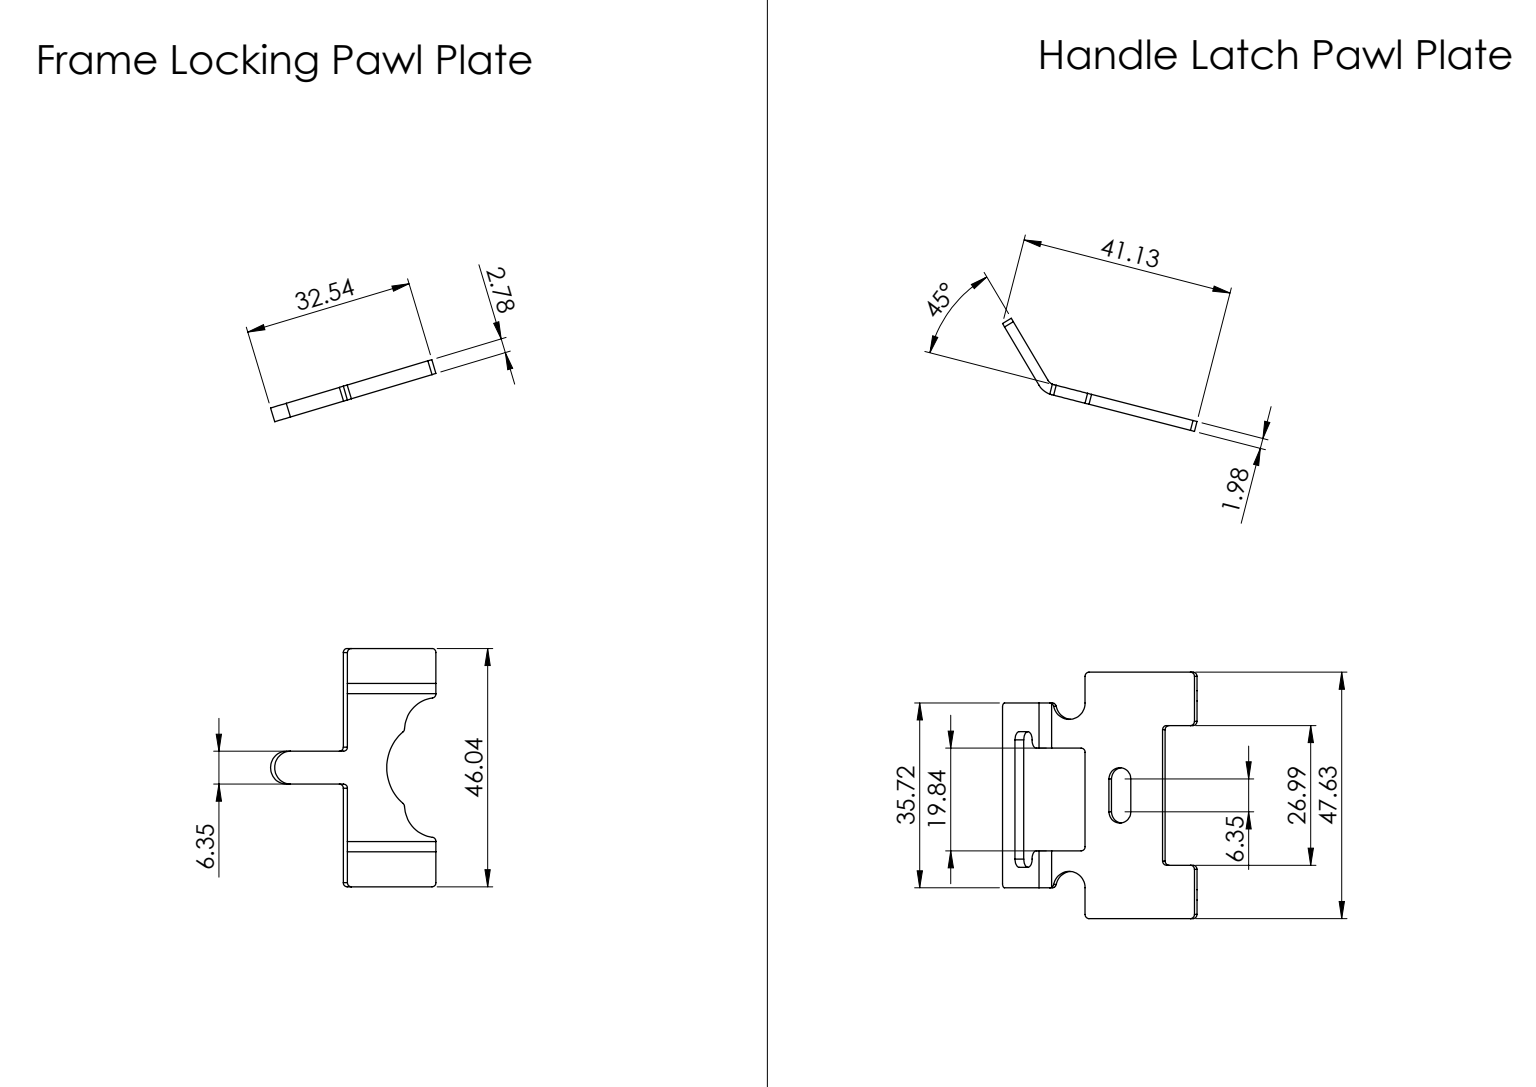
ISO-10303-21;
HEADER;
FILE_DESCRIPTION (('STEP AP214'),
    '1' );
FILE_NAME ('Frame Locking Pawl Plate.step',
    '2026-10-09T14:10:49',
    ( '' ),
    ( '' ),
    'SwSTEP 2.0',
    'SolidWorks 2026',
    '' );
FILE_SCHEMA (( 'AUTOMOTIVE_DESIGN' ));
ENDSEC;

DATA;
#12=VECTOR ( 'NONE', #9469, 1000.000000000000227 ) ;
#61=CARTESIAN_POINT ( 'NONE',  ( 14.43917063414567536, -6.754812500000002551, 2.343183994106907697 ) ) ;
#87=ORIENTED_EDGE ( 'NONE', *, *, #3995, .F. ) ;
#93=VERTEX_POINT ( 'NONE', #19156 ) ;
#123=DIRECTION ( 'NONE',  ( 0.2868778675745011220, 0.000000000000000000, 0.9579671649362034858 ) ) ;
#130=CARTESIAN_POINT ( 'NONE',  ( 13.67756757867809725, 20.23395749999999893, 2.571257636385987144 ) ) ;
#285=ORIENTED_EDGE ( 'NONE', *, *, #4081, .F. ) ;
#292=CARTESIAN_POINT ( 'NONE',  ( 29.98909767165928386, 30.50833916023545811, -5.214162619065493054 ) ) ;
#304=VERTEX_POINT ( 'NONE', #16295 ) ;
#353=DIRECTION ( 'NONE',  ( 0.000000000000000000, -1.000000000000000000, 0.000000000000000000 ) ) ;
#357=VECTOR ( 'NONE', #20266, 1000.000000000000000 ) ;
#367=VERTEX_POINT ( 'NONE', #5509 ) ;
#389=EDGE_CURVE ( 'NONE', #18438, #18286, #10607, .T. ) ;
#413=LINE ( 'NONE', #20514, #19877 ) ;
#419=EDGE_CURVE ( 'NONE', #13188, #14728, #15986, .T. ) ;
#453=ADVANCED_FACE ( 'NONE', ( #15932 ), #20761, .T. ) ;
#500=CARTESIAN_POINT ( 'NONE',  ( 13.67756757867809725, 38.48766750000000059, 2.571257636385987144 ) ) ;
#503=VECTOR ( 'NONE', #5511, 1000.000000000000227 ) ;
#522=CARTESIAN_POINT ( 'NONE',  ( 14.43917063414567536, 39.28268749999999443, 2.343183994106907697 ) ) ;
#539=VERTEX_POINT ( 'NONE', #21310 ) ;
#544=EDGE_CURVE ( 'NONE', #7495, #1968, #3265, .T. ) ;
#640=ORIENTED_EDGE ( 'NONE', *, *, #20179, .T. ) ;
#679=DIRECTION ( 'NONE',  ( 0.2868778675745011220, 0.000000000000000000, 0.9579671649362033747 ) ) ;
#697=LINE ( 'NONE', #19041, #16642 ) ;
#699=VERTEX_POINT ( 'NONE', #3620 ) ;
#749=ORIENTED_EDGE ( 'NONE', *, *, #21150, .T. ) ;
#760=DIRECTION ( 'NONE',  ( 0.000000000000000000, -1.000000000000000000, 0.000000000000000000 ) ) ;
#775=LINE ( 'NONE', #19445, #8515 ) ;
#847=CARTESIAN_POINT ( 'NONE',  ( 13.67756757867809725, -5.959792500000001603, 2.571257636385987144 ) ) ;
#868=ADVANCED_FACE ( 'NONE', ( #18966 ), #7371, .T. ) ;
#886=CARTESIAN_POINT ( 'NONE',  ( 29.98909767165928386, 39.28268749999999443, -5.214162619065493054 ) ) ;
#891=ORIENTED_EDGE ( 'NONE', *, *, #18599, .F. ) ;
#912=DIRECTION ( 'NONE',  ( 0.000000000000000000, 1.000000000000000000, 0.000000000000000000 ) ) ;
#944=DIRECTION ( 'NONE',  ( -0.2868778675745011220, 0.000000000000000000, -0.9579671649362034858 ) ) ;
#961=ORIENTED_EDGE ( 'NONE', *, *, #2073, .T. ) ;
#980=ORIENTED_EDGE ( 'NONE', *, *, #6673, .F. ) ;
#983=APPLICATION_CONTEXT ( 'automotive_design' ) ;
#996=CARTESIAN_POINT ( 'NONE',  ( 24.43309469626978725, 23.18727947754285879, -0.6496488801123181389 ) ) ;
#1024=LINE ( 'NONE', #4465, #19918 ) ;
#1049=FACE_OUTER_BOUND ( 'NONE', #12036, .T. ) ;
#1092=DIRECTION ( 'NONE',  ( 0.9579671649362032637, 0.000000000000000000, -0.2868778675745011775 ) ) ;
#1103=ORIENTED_EDGE ( 'NONE', *, *, #19401, .T. ) ;
#1104=DIRECTION ( 'NONE',  ( 0.9579671649362032637, 0.000000000000000000, -0.2868778675745010664 ) ) ;
#1115=EDGE_CURVE ( 'NONE', #20009, #20529, #13174, .T. ) ;
#1149=CARTESIAN_POINT ( 'NONE',  ( 29.22749461619170219, -6.754812500000002551, -4.986088976786413163 ) ) ;
#1157=ORIENTED_EDGE ( 'NONE', *, *, #8283, .T. ) ;
#1165=CARTESIAN_POINT ( 'NONE',  ( 30.78626241496060700, 30.50833916023545811, -2.552201779827368622 ) ) ;
#1191=ORIENTED_EDGE ( 'NONE', *, *, #8598, .F. ) ;
#1305=CARTESIAN_POINT ( 'NONE',  ( 13.67756757867809725, 0.001587500000000546807, 2.571257636385987144 ) ) ;
#1317=ORIENTED_EDGE ( 'NONE', *, *, #20399, .T. ) ;
#1328=CARTESIAN_POINT ( 'NONE',  ( 30.02465935949302533, 30.50833916023545811, -2.324128137548288731 ) ) ;
#1348=DIRECTION ( 'NONE',  ( 0.2868778675745011220, 0.000000000000000000, 0.9579671649362034858 ) ) ;
#1401=DIRECTION ( 'NONE',  ( 0.000000000000000000, -1.000000000000000000, 0.000000000000000000 ) ) ;
#1450=MECHANICAL_DESIGN_GEOMETRIC_PRESENTATION_REPRESENTATION('',(#2514),#7809);
#1483=AXIS2_PLACEMENT_3D ( 'NONE', #17356, #2200, #12384 ) ;
#1499=VERTEX_POINT ( 'NONE', #1305 ) ;
#1504=ORIENTED_EDGE ( 'NONE', *, *, #10980, .T. ) ;
#1583=DIRECTION ( 'NONE',  ( 0.2868778675745011220, 0.000000000000000000, 0.9579671649362034858 ) ) ;
#1586=ORIENTED_EDGE ( 'NONE', *, *, #5324, .F. ) ;
#1594=EDGE_LOOP ( 'NONE', ( #10062, #8009, #14700, #9478, #16584, #21246 ) ) ;
#1614=DIRECTION ( 'NONE',  ( 0.000000000000000000, 1.000000000000000000, 0.000000000000000000 ) ) ;
#1616=PLANE ( 'NONE',  #9906 ) ;
#1628=DIRECTION ( 'NONE',  ( 0.9579671649362032637, 0.000000000000000000, -0.2868778675745012885 ) ) ;
#1666=DIRECTION ( 'NONE',  ( -0.2868778675745011220, 0.000000000000000000, -0.9579671649362034858 ) ) ;
#1678=LINE ( 'NONE', #15312, #7096 ) ;
#1696=AXIS2_PLACEMENT_3D ( 'NONE', #16112, #944, #14450 ) ;
#1743=EDGE_LOOP ( 'NONE', ( #7465, #6376, #15613, #2042 ) ) ;
#1791=ORIENTED_EDGE ( 'NONE', *, *, #11880, .T. ) ;
#1847=DIRECTION ( 'NONE',  ( 0.000000000000000000, 1.000000000000000000, 0.000000000000000000 ) ) ;
#1883=EDGE_CURVE ( 'NONE', #20529, #15912, #413, .T. ) ;
#1968=VERTEX_POINT ( 'NONE', #9028 ) ;
#1980=CYLINDRICAL_SURFACE ( 'NONE', #5566, 8.929687500000001776 ) ;
#1986=ORIENTED_EDGE ( 'NONE', *, *, #8283, .F. ) ;
#1991=ORIENTED_EDGE ( 'NONE', *, *, #5836, .T. ) ;
#2037=DIRECTION ( 'NONE',  ( -0.9579671649362032637, 0.000000000000000000, 0.2868778675745010664 ) ) ;
#2041=VECTOR ( 'NONE', #20727, 1000.000000000000227 ) ;
#2042=ORIENTED_EDGE ( 'NONE', *, *, #14952, .T. ) ;
#2056=AXIS2_PLACEMENT_3D ( 'NONE', #11844, #18251, #3220 ) ;
#2073=EDGE_CURVE ( 'NONE', #18658, #16568, #9570, .T. ) ;
#2075=CARTESIAN_POINT ( 'NONE',  ( 12.91596452321051558, 20.23395749999999893, 2.799331278665067479 ) ) ;
#2131=FILL_AREA_STYLE ('',( #8988 ) ) ;
#2168=CARTESIAN_POINT ( 'NONE',  ( 2.651964239740473683, 19.43893749999999798, 5.873042593501262232 ) ) ;
#2182=EDGE_LOOP ( 'NONE', ( #7820, #21657, #6898, #18046 ) ) ;
#2200=DIRECTION ( 'NONE',  ( -0.2868778675745011220, 0.000000000000000000, -0.9579671649362034858 ) ) ;
#2230=CARTESIAN_POINT ( 'NONE',  ( 17.85969298310271114, 32.52628750000000224, 1.318856445756055873 ) ) ;
#2234=AXIS2_PLACEMENT_3D ( 'NONE', #14022, #2275, #17644 ) ;
#2244=VECTOR ( 'NONE', #14358, 1000.000000000000227 ) ;
#2254=ORIENTED_EDGE ( 'NONE', *, *, #6519, .T. ) ;
#2275=DIRECTION ( 'NONE',  ( 0.000000000000000000, 0.000000000000000000, 1.000000000000000000 ) ) ;
#2309=CARTESIAN_POINT ( 'NONE',  ( 14.43917063414567536, 39.28268749999999443, 2.343183994106907697 ) ) ;
#2314=EDGE_LOOP ( 'NONE', ( #18332, #4923, #10343, #5168 ) ) ;
#2324=CARTESIAN_POINT ( 'NONE',  ( 1.854799496439154316, 16.26393749999999727, 3.211081754263136911 ) ) ;
#2329=DIRECTION ( 'NONE',  ( -0.9579671649362030417, 0.000000000000000000, 0.2868778675745017326 ) ) ;
#2377=ORIENTED_EDGE ( 'NONE', *, *, #3048, .F. ) ;
#2406=CARTESIAN_POINT ( 'NONE',  ( 13.67756757867809725, 38.48766750000000059, 2.571257636385987144 ) ) ;
#2408=ORIENTED_EDGE ( 'NONE', *, *, #389, .F. ) ;
#2416=ORIENTED_EDGE ( 'NONE', *, *, #15750, .T. ) ;
#2471=SURFACE_STYLE_USAGE ( .BOTH. , #15984 ) ;
#2514=STYLED_ITEM ( 'NONE', ( #13999 ), #6428 ) ;
#2517=ORIENTED_EDGE ( 'NONE', *, *, #9221, .T. ) ;
#2553=AXIS2_PLACEMENT_3D ( 'NONE', #9600, #19557, #18127 ) ;
#2573=CARTESIAN_POINT ( 'NONE',  ( 30.78626241496060700, -5.959792500000001603, -2.552201779827368622 ) ) ;
#2602=EDGE_LOOP ( 'NONE', ( #11906, #1791, #11117, #1103 ) ) ;
#2617=ORIENTED_EDGE ( 'NONE', *, *, #8323, .F. ) ;
#2623=CARTESIAN_POINT ( 'NONE',  ( 29.03861462519914838, 16.26393749999999727, -4.929525984831418128 ) ) ;
#2642=ORIENTED_EDGE ( 'NONE', *, *, #15646, .F. ) ;
#2646=PLANE ( 'NONE',  #13935 ) ;
#2695=DIRECTION ( 'NONE',  ( 0.6050250551579484659, -0.7753173868113210077, -0.1811839737371541414 ) ) ;
#2707=CARTESIAN_POINT ( 'NONE',  ( 30.78626241496060700, 30.54508749999999750, -2.552201779827368622 ) ) ;
#2733=CARTESIAN_POINT ( 'NONE',  ( 1.854799496439154316, 19.43893749999999798, 3.211081754263136911 ) ) ;
#2741=EDGE_LOOP ( 'NONE', ( #14917, #640, #16235, #11591 ) ) ;
#2751=AXIS2_PLACEMENT_3D ( 'NONE', #1328, #21561, #13077 ) ;
#2752=EDGE_LOOP ( 'NONE', ( #2617, #17130, #21168, #2517, #13607, #11181 ) ) ;
#2754=CARTESIAN_POINT ( 'NONE',  ( 30.78626241496060700, 30.50833916023545811, -2.552201779827368622 ) ) ;
#2793=CYLINDRICAL_SURFACE ( 'NONE', #8442, 6.350000000000001421 ) ;
#2804=FACE_OUTER_BOUND ( 'NONE', #2847, .T. ) ;
#2834=VECTOR ( 'NONE', #18906, 1000.000000000000000 ) ;
#2843=LINE ( 'NONE', #2733, #12 ) ;
#2847=EDGE_LOOP ( 'NONE', ( #13729, #21082, #4101, #13970 ) ) ;
#2857=CARTESIAN_POINT ( 'NONE',  ( 12.91596452321051558, 12.29391749999999739, 2.799331278665067479 ) ) ;
#2875=CARTESIAN_POINT ( 'NONE',  ( 30.10940225190841701, 2.809619014187358932, -2.349505688218141319 ) ) ;
#2888=CARTESIAN_POINT ( 'NONE',  ( 29.98909767165928386, 38.48766750000000059, -5.214162619065493054 ) ) ;
#2895=CARTESIAN_POINT ( 'NONE',  ( 1.854799496439154316, 13.08893749999999834, 3.211081754263136911 ) ) ;
#2941=EDGE_LOOP ( 'NONE', ( #9817, #8604, #12640, #18611 ) ) ;
#2999=ADVANCED_FACE ( 'NONE', ( #11044 ), #2646, .T. ) ;
#3048=EDGE_CURVE ( 'NONE', #12509, #19832, #7231, .T. ) ;
#3169=VERTEX_POINT ( 'NONE', #8888 ) ;
#3182=ADVANCED_FACE ( 'NONE', ( #11587 ), #7010, .T. ) ;
#3220=DIRECTION ( 'NONE',  ( 0.9579671649362032637, 0.000000000000000000, -0.2868778675745011775 ) ) ;
#3233=FACE_OUTER_BOUND ( 'NONE', #1743, .T. ) ;
#3237=VECTOR ( 'NONE', #912, 1000.000000000000000 ) ;
#3265=CIRCLE ( 'NONE', #20890, 0.7950200000000005041 ) ;
#3291=FACE_OUTER_BOUND ( 'NONE', #2741, .T. ) ;
#3351=PLANE ( 'NONE',  #18829 ) ;
#3353=LINE ( 'NONE', #15082, #4579 ) ;
#3449=FACE_OUTER_BOUND ( 'NONE', #8597, .T. ) ;
#3511=ORIENTED_EDGE ( 'NONE', *, *, #20455, .T. ) ;
#3516=CARTESIAN_POINT ( 'NONE',  ( 12.11879977990919421, 19.43893749999999798, 0.1373704394269426865 ) ) ;
#3519=VERTEX_POINT ( 'NONE', #1149 ) ;
#3545=LINE ( 'NONE', #10282, #13496 ) ;
#3585=ADVANCED_FACE ( 'NONE', ( #18487 ), #20127, .F. ) ;
#3599=EDGE_LOOP ( 'NONE', ( #7691, #17588, #10865, #20840 ) ) ;
#3614=VECTOR ( 'NONE', #20424, 1000.000000000000000 ) ;
#3618=ORIENTED_EDGE ( 'NONE', *, *, #20772, .T. ) ;
#3620=CARTESIAN_POINT ( 'NONE',  ( 12.88040283537677588, 12.29391749999999739, -0.09070320285213756550 ) ) ;
#3624=LINE ( 'NONE', #13805, #21432 ) ;
#3636=ORIENTED_EDGE ( 'NONE', *, *, #13339, .F. ) ;
#3644=ORIENTED_EDGE ( 'NONE', *, *, #13978, .F. ) ;
#3653=CARTESIAN_POINT ( 'NONE',  ( 22.04181838752732148, 16.26393749999999727, 0.06645525512612464325 ) ) ;
#3656=ORIENTED_EDGE ( 'NONE', *, *, #15060, .T. ) ;
#3734=DIRECTION ( 'NONE',  ( 0.9579671649362032637, 0.000000000000000000, -0.2868778675745013440 ) ) ;
#3818=ORIENTED_EDGE ( 'NONE', *, *, #1115, .F. ) ;
#3826=CARTESIAN_POINT ( 'NONE',  ( 29.83577936850046441, 16.26393749999999727, -2.267565145593293696 ) ) ;
#3842=DIRECTION ( 'NONE',  ( 0.2868778675745011220, 0.000000000000000000, 0.9579671649362034858 ) ) ;
#3900=CIRCLE ( 'NONE', #18402, 0.7950200000000005041 ) ;
#3920=ORIENTED_EDGE ( 'NONE', *, *, #389, .T. ) ;
#3950=CARTESIAN_POINT ( 'NONE',  ( 12.91596452321051558, 19.43893749999999798, 2.799331278665067479 ) ) ;
#3951=DIRECTION ( 'NONE',  ( 0.9579671649362032637, 0.000000000000000000, -0.2868778675745010664 ) ) ;
#3960=ORIENTED_EDGE ( 'NONE', *, *, #4201, .F. ) ;
#3971=AXIS2_PLACEMENT_3D ( 'NONE', #19107, #7394, #14165 ) ;
#3995=EDGE_CURVE ( 'NONE', #4404, #11521, #17573, .T. ) ;
#4046=CARTESIAN_POINT ( 'NONE',  ( 12.88040283537677588, 20.23395749999999893, -0.09070320285213756550 ) ) ;
#4067=DIRECTION ( 'NONE',  ( -0.2868778675745010664, 0.000000000000000000, -0.9579671649362032637 ) ) ;
#4081=EDGE_CURVE ( 'NONE', #15859, #10888, #8991, .T. ) ;
#4101=ORIENTED_EDGE ( 'NONE', *, *, #6921, .T. ) ;
#4128=( NAMED_UNIT ( * ) SI_UNIT ( $, .STERADIAN. ) SOLID_ANGLE_UNIT ( ) );
#4131=CIRCLE ( 'NONE', #12241, 3.175000000000000711 ) ;
#4136=ADVANCED_FACE ( 'NONE', ( #14606 ), #21647, .T. ) ;
#4144=UNCERTAINTY_MEASURE_WITH_UNIT (LENGTH_MEASURE( 1.000000000000000082E-05 ), #9340, 'distance_accuracy_value', 'NONE');
#4146=CIRCLE ( 'NONE', #16510, 8.929687500000000000 ) ;
#4186=CIRCLE ( 'NONE', #2056, 0.7950200000000011702 ) ;
#4201=EDGE_CURVE ( 'NONE', #17126, #19423, #15035, .T. ) ;
#4238=ORIENTED_EDGE ( 'NONE', *, *, #18010, .F. ) ;
#4285=LINE ( 'NONE', #2406, #14814 ) ;
#4305=DIRECTION ( 'NONE',  ( -0.1065921516619563053, -0.9937903127262235348, 0.03192064434796804129 ) ) ;
#4329=VECTOR ( 'NONE', #20195, 1000.000000000000227 ) ;
#4353=ORIENTED_EDGE ( 'NONE', *, *, #10760, .T. ) ;
#4404=VERTEX_POINT ( 'NONE', #18434 ) ;
#4415=AXIS2_PLACEMENT_3D ( 'NONE', #13870, #18919, #353 ) ;
#4432=DIRECTION ( 'NONE',  ( 0.000000000000000000, 1.000000000000000000, 0.000000000000000000 ) ) ;
#4438=DIRECTION ( 'NONE',  ( -0.9579671649362033747, 0.000000000000000000, 0.2868778675745011220 ) ) ;
#4465=CARTESIAN_POINT ( 'NONE',  ( 12.11879977990919421, 19.43893749999999798, 0.1373704394269426865 ) ) ;
#4470=DIRECTION ( 'NONE',  ( 0.000000000000000000, 1.000000000000000000, 0.000000000000000000 ) ) ;
#4487=PLANE ( 'NONE',  #4539 ) ;
#4498=ORIENTED_EDGE ( 'NONE', *, *, #21150, .F. ) ;
#4518=CARTESIAN_POINT ( 'NONE',  ( 29.98909767165928386, -6.754812500000002551, -5.214162619065493054 ) ) ;
#4535=EDGE_CURVE ( 'NONE', #699, #15950, #5127, .T. ) ;
#4539=AXIS2_PLACEMENT_3D ( 'NONE', #9015, #11336, #8338 ) ;
#4543=LINE ( 'NONE', #19781, #12358 ) ;
#4574=LINE ( 'NONE', #19602, #14602 ) ;
#4579=VECTOR ( 'NONE', #13637, 1000.000000000000227 ) ;
#4584=VERTEX_POINT ( 'NONE', #522 ) ;
#4597=VERTEX_POINT ( 'NONE', #19604 ) ;
#4627=CARTESIAN_POINT ( 'NONE',  ( 23.15492293361681320, 8.724202693596797786, -3.167564836549936480 ) ) ;
#4652=AXIS2_PLACEMENT_3D ( 'NONE', #14182, #10736, #7305 ) ;
#4673=ORIENTED_EDGE ( 'NONE', *, *, #6673, .T. ) ;
#4682=DIRECTION ( 'NONE',  ( 0.2868778675745010664, 0.000000000000000000, 0.9579671649362032637 ) ) ;
#4707=EDGE_LOOP ( 'NONE', ( #3960, #4238, #8843, #749 ) ) ;
#4738=CYLINDRICAL_SURFACE ( 'NONE', #10361, 0.7950200000000005041 ) ;
#4753=ORIENTED_EDGE ( 'NONE', *, *, #9918, .T. ) ;
#4759=VERTEX_POINT ( 'NONE', #9756 ) ;
#4772=ORIENTED_EDGE ( 'NONE', *, *, #16413, .T. ) ;
#4774=DIRECTION ( 'NONE',  ( 0.000000000000000000, -1.000000000000000000, 0.000000000000000000 ) ) ;
#4810=DIRECTION ( 'NONE',  ( -0.2868778675745010664, 0.000000000000000000, -0.9579671649362032637 ) ) ;
#4898=EDGE_CURVE ( 'NONE', #699, #19423, #17273, .T. ) ;
#4919=CARTESIAN_POINT ( 'NONE',  ( 24.99127163628573456, 23.80367230640320031, 2.964528152719008158 ) ) ;
#4923=ORIENTED_EDGE ( 'NONE', *, *, #20455, .F. ) ;
#4958=ORIENTED_EDGE ( 'NONE', *, *, #4081, .T. ) ;
#5019=ORIENTED_EDGE ( 'NONE', *, *, #5849, .F. ) ;
#5022=AXIS2_PLACEMENT_3D ( 'NONE', #4919, #11559, #11458 ) ;
#5039=CARTESIAN_POINT ( 'NONE',  ( 30.78626241496060700, 2.019535839764540430, -2.552201779827368622 ) ) ;
#5042=CIRCLE ( 'NONE', #14600, 0.7950199999999993938 ) ;
#5089=CARTESIAN_POINT ( 'NONE',  ( 29.03861462519914838, 16.26393749999999727, -4.929525984831418128 ) ) ;
#5095=DIRECTION ( 'NONE',  ( -0.2868778675745010664, 0.000000000000000000, -0.9579671649362032637 ) ) ;
#5099=ORIENTED_EDGE ( 'NONE', *, *, #8046, .F. ) ;
#5127=CIRCLE ( 'NONE', #15398, 0.7950199999999993938 ) ;
#5168=ORIENTED_EDGE ( 'NONE', *, *, #6705, .F. ) ;
#5182=CARTESIAN_POINT ( 'NONE',  ( 24.71252020198295085, 8.768263569673496960, -0.7333271064221494884 ) ) ;
#5299=DIRECTION ( 'NONE',  ( 0.9579671649362032637, 0.000000000000000000, -0.2868778675745010664 ) ) ;
#5324=EDGE_CURVE ( 'NONE', #9688, #15950, #18352, .T. ) ;
#5353=DIRECTION ( 'NONE',  ( -0.9579671649362033747, 0.000000000000000000, 0.2868778675745011220 ) ) ;
#5379=AXIS2_PLACEMENT_3D ( 'NONE', #3826, #8677, #15451 ) ;
#5391=CARTESIAN_POINT ( 'NONE',  ( 14.43917063414567536, 38.48766750000000059, 2.343183994106907697 ) ) ;
#5404=DIRECTION ( 'NONE',  ( 0.9579671649362033747, 0.000000000000000000, -0.2868778675745010664 ) ) ;
#5437=CARTESIAN_POINT ( 'NONE',  ( 14.43917063414567536, -6.754812500000002551, 2.343183994106907697 ) ) ;
#5485=LINE ( 'NONE', #7161, #7416 ) ;
#5488=ORIENTED_EDGE ( 'NONE', *, *, #6705, .T. ) ;
#5509=CARTESIAN_POINT ( 'NONE',  ( 13.67756757867809725, -5.959792500000001603, 2.571257636385987144 ) ) ;
#5511=DIRECTION ( 'NONE',  ( -0.2868778675745010664, 0.000000000000000000, -0.9579671649362032637 ) ) ;
#5515=ORIENTED_EDGE ( 'NONE', *, *, #16413, .F. ) ;
#5539=DIRECTION ( 'NONE',  ( 0.9579671649362032637, 0.000000000000000000, -0.2868778675745010664 ) ) ;
#5546=DIRECTION ( 'NONE',  ( 0.2868778675745010664, 0.000000000000000000, 0.9579671649362032637 ) ) ;
#5555=ORIENTED_EDGE ( 'NONE', *, *, #17087, .T. ) ;
#5566=AXIS2_PLACEMENT_3D ( 'NONE', #5089, #8720, #5404 ) ;
#5639=VERTEX_POINT ( 'NONE', #19117 ) ;
#5676=AXIS2_PLACEMENT_3D ( 'NONE', #21844, #13355, #1614 ) ;
#5742=EDGE_CURVE ( 'NONE', #18438, #4597, #6077, .T. ) ;
#5780=ORIENTED_EDGE ( 'NONE', *, *, #11880, .F. ) ;
#5836=EDGE_CURVE ( 'NONE', #12549, #304, #20532, .T. ) ;
#5849=EDGE_CURVE ( 'NONE', #6840, #93, #20183, .T. ) ;
#5885=DIRECTION ( 'NONE',  ( 0.9579671649362033747, 0.000000000000000000, -0.2868778675745010664 ) ) ;
#6022=CYLINDRICAL_SURFACE ( 'NONE', #9479, 0.7950200000000003930 ) ;
#6077=CIRCLE ( 'NONE', #7848, 0.7950200000000011702 ) ;
#6081=ADVANCED_FACE ( 'NONE', ( #10112 ), #19843, .T. ) ;
#6106=ORIENTED_EDGE ( 'NONE', *, *, #6925, .T. ) ;
#6117=DIRECTION ( 'NONE',  ( 0.9579671649362033747, 0.000000000000000000, -0.2868778675745010664 ) ) ;
#6230=ORIENTED_EDGE ( 'NONE', *, *, #11251, .T. ) ;
#6244=LINE ( 'NONE', #6352, #10771 ) ;
#6260=ORIENTED_EDGE ( 'NONE', *, *, #4201, .T. ) ;
#6306=DIRECTION ( 'NONE',  ( 0.2868778675745011220, 0.000000000000000000, 0.9579671649362034858 ) ) ;
#6352=CARTESIAN_POINT ( 'NONE',  ( 29.22749461619170219, 39.28268749999999443, -4.986088976786413163 ) ) ;
#6376=ORIENTED_EDGE ( 'NONE', *, *, #19723, .F. ) ;
#6379=VECTOR ( 'NONE', #10460, 1000.000000000000227 ) ;
#6396=DIRECTION ( 'NONE',  ( 0.000000000000000000, -1.000000000000000000, 0.000000000000000000 ) ) ;
#6428=MANIFOLD_SOLID_BREP ( 'Stock-MAS-676-1', #9231 ) ;
#6448=AXIS2_PLACEMENT_3D ( 'NONE', #16744, #1583, #8327 ) ;
#6509=PRODUCT ( 'Frame Locking Pawl Plate', 'Frame Locking Pawl Plate', '', ( #20468 ) ) ;
#6519=EDGE_CURVE ( 'NONE', #18557, #3519, #697, .T. ) ;
#6562=PLANE ( 'NONE',  #7154 ) ;
#6588=ORIENTED_EDGE ( 'NONE', *, *, #544, .F. ) ;
#6599=ORIENTED_EDGE ( 'NONE', *, *, #3048, .T. ) ;
#6610=LINE ( 'NONE', #13593, #8886 ) ;
#6632=LINE ( 'NONE', #13622, #18426 ) ;
#6673=EDGE_CURVE ( 'NONE', #12549, #17651, #8204, .T. ) ;
#6700=CARTESIAN_POINT ( 'NONE',  ( 12.88040283537677588, -6.754812500000002551, -0.09070320285213756550 ) ) ;
#6703=ADVANCED_FACE ( 'NONE', ( #16925 ), #13633, .T. ) ;
#6705=EDGE_CURVE ( 'NONE', #7786, #17651, #16266, .T. ) ;
#6706=ADVANCED_FACE ( 'NONE', ( #3233 ), #16615, .T. ) ;
#6726=PLANE ( 'NONE',  #12969 ) ;
#6822=CIRCLE ( 'NONE', #10718, 0.7950199999999993938 ) ;
#6840=VERTEX_POINT ( 'NONE', #13737 ) ;
#6852=ADVANCED_FACE ( 'NONE', ( #20668 ), #9063, .T. ) ;
#6885=DIRECTION ( 'NONE',  ( 0.000000000000000000, -1.000000000000000000, 0.000000000000000000 ) ) ;
#6897=DIRECTION ( 'NONE',  ( 0.000000000000000000, 1.000000000000000000, 0.000000000000000000 ) ) ;
#6898=ORIENTED_EDGE ( 'NONE', *, *, #15391, .F. ) ;
#6921=EDGE_CURVE ( 'NONE', #7865, #6840, #15407, .T. ) ;
#6925=EDGE_CURVE ( 'NONE', #10936, #5639, #14073, .T. ) ;
#6949=ADVANCED_FACE ( 'NONE', ( #10410 ), #17152, .T. ) ;
#6962=LINE ( 'NONE', #20004, #11377 ) ;
#7010=PLANE ( 'NONE',  #16065 ) ;
#7042=EDGE_CURVE ( 'NONE', #539, #7495, #17819, .T. ) ;
#7096=VECTOR ( 'NONE', #15195, 1000.000000000000227 ) ;
#7132=AXIS2_PLACEMENT_3D ( 'NONE', #3653, #13838, #17141 ) ;
#7137=DIRECTION ( 'NONE',  ( -0.2868778675745011220, 0.000000000000000000, -0.9579671649362034858 ) ) ;
#7148=LINE ( 'NONE', #15230, #16299 ) ;
#7154=AXIS2_PLACEMENT_3D ( 'NONE', #18068, #9542, #14665 ) ;
#7161=CARTESIAN_POINT ( 'NONE',  ( 12.11879977990919421, 13.08893749999999834, 0.1373704394269426865 ) ) ;
#7207=ORIENTED_EDGE ( 'NONE', *, *, #18883, .F. ) ;
#7231=CIRCLE ( 'NONE', #19574, 6.350000000000002309 ) ;
#7262=ORIENTED_EDGE ( 'NONE', *, *, #15391, .T. ) ;
#7305=DIRECTION ( 'NONE',  ( 0.9564948366894089338, 0.05542109139015086172, -0.2864369564417716951 ) ) ;
#7322=FACE_OUTER_BOUND ( 'NONE', #1594, .T. ) ;
#7350=ORIENTED_EDGE ( 'NONE', *, *, #19779, .F. ) ;
#7359=DIRECTION ( 'NONE',  ( 0.2868778675745011220, 0.000000000000000000, 0.9579671649362033747 ) ) ;
#7371=PLANE ( 'NONE',  #17029 ) ;
#7394=DIRECTION ( 'NONE',  ( -0.2868778675745011220, 0.000000000000000000, -0.9579671649362034858 ) ) ;
#7407=DIRECTION ( 'NONE',  ( 0.000000000000000000, 1.000000000000000000, 0.000000000000000000 ) ) ;
#7416=VECTOR ( 'NONE', #10244, 1000.000000000000227 ) ;
#7465=ORIENTED_EDGE ( 'NONE', *, *, #5742, .F. ) ;
#7495=VERTEX_POINT ( 'NONE', #19186 ) ;
#7501=ORIENTED_EDGE ( 'NONE', *, *, #13815, .F. ) ;
#7557=CARTESIAN_POINT ( 'NONE',  ( 29.98909767165928386, 2.019535839764540430, -5.214162619065493054 ) ) ;
#7564=EDGE_LOOP ( 'NONE', ( #14812, #18530, #3818, #4353 ) ) ;
#7577=ORIENTED_EDGE ( 'NONE', *, *, #15750, .F. ) ;
#7589=CARTESIAN_POINT ( 'NONE',  ( 12.11879977990919421, 13.08893749999999834, 0.1373704394269426865 ) ) ;
#7633=DIRECTION ( 'NONE',  ( 0.2868778675745010664, 0.000000000000000000, 0.9579671649362032637 ) ) ;
#7666=DIRECTION ( 'NONE',  ( 0.2868778675745011220, 0.000000000000000000, 0.9579671649362034858 ) ) ;
#7691=ORIENTED_EDGE ( 'NONE', *, *, #9143, .T. ) ;
#7704=ORIENTED_EDGE ( 'NONE', *, *, #4898, .T. ) ;
#7738=ORIENTED_EDGE ( 'NONE', *, *, #8968, .T. ) ;
#7741=VECTOR ( 'NONE', #8594, 1000.000000000000227 ) ;
#7786=VERTEX_POINT ( 'NONE', #16342 ) ;
#7802=VECTOR ( 'NONE', #9794, 1000.000000000000000 ) ;
#7809=( GEOMETRIC_REPRESENTATION_CONTEXT ( 3 ) GLOBAL_UNCERTAINTY_ASSIGNED_CONTEXT ( ( #12116 ) ) GLOBAL_UNIT_ASSIGNED_CONTEXT ( ( #10539, #17177, #4128 ) ) REPRESENTATION_CONTEXT ( 'NONE', 'WORKASPACE' ) );
#7820=ORIENTED_EDGE ( 'NONE', *, *, #12450, .T. ) ;
#7830=AXIS2_PLACEMENT_3D ( 'NONE', #8160, #14938, #1628 ) ;
#7832=ORIENTED_EDGE ( 'NONE', *, *, #6921, .F. ) ;
#7848=AXIS2_PLACEMENT_3D ( 'NONE', #16366, #21427, #1092 ) ;
#7865=VERTEX_POINT ( 'NONE', #21626 ) ;
#7960=EDGE_CURVE ( 'NONE', #5639, #14728, #19153, .T. ) ;
#8009=ORIENTED_EDGE ( 'NONE', *, *, #12944, .T. ) ;
#8017=ORIENTED_EDGE ( 'NONE', *, *, #5836, .F. ) ;
#8044=DIRECTION ( 'NONE',  ( -0.2868778675745011220, 0.000000000000000000, -0.9579671649362034858 ) ) ;
#8046=EDGE_CURVE ( 'NONE', #9688, #539, #10121, .T. ) ;
#8051=DIRECTION ( 'NONE',  ( 0.000000000000000000, 1.000000000000000000, 0.000000000000000000 ) ) ;
#8077=ORIENTED_EDGE ( 'NONE', *, *, #419, .F. ) ;
#8100=CARTESIAN_POINT ( 'NONE',  ( 30.78626241496060700, 38.48766750000000059, -2.552201779827368622 ) ) ;
#8116=AXIS2_PLACEMENT_3D ( 'NONE', #16863, #7137, #13906 ) ;
#8123=VECTOR ( 'NONE', #15838, 1000.000000000000227 ) ;
#8152=CARTESIAN_POINT ( 'NONE',  ( 12.88040283537677588, 39.28268749999999443, -0.09070320285213756550 ) ) ;
#8157=ORIENTED_EDGE ( 'NONE', *, *, #9944, .F. ) ;
#8160=CARTESIAN_POINT ( 'NONE',  ( 11.07961582054159244, 12.29391749999999739, -3.332761710603877159 ) ) ;
#8204=LINE ( 'NONE', #11853, #14509 ) ;
#8271=LINE ( 'NONE', #21757, #4329 ) ;
#8283=EDGE_CURVE ( 'NONE', #19832, #10623, #9941, .T. ) ;
#8292=LINE ( 'NONE', #15064, #14421 ) ;
#8323=EDGE_CURVE ( 'NONE', #1499, #3169, #3545, .T. ) ;
#8327=DIRECTION ( 'NONE',  ( 0.9579671649362033747, 0.000000000000000000, -0.2868778675745011775 ) ) ;
#8338=DIRECTION ( 'NONE',  ( -0.2868778675745010664, 0.000000000000000000, -0.9579671649362032637 ) ) ;
#8339=LINE ( 'NONE', #13440, #20986 ) ;
#8374=ORIENTED_EDGE ( 'NONE', *, *, #17598, .T. ) ;
#8390=EDGE_CURVE ( 'NONE', #16118, #12232, #775, .T. ) ;
#8405=CARTESIAN_POINT ( 'NONE',  ( 21.24465364422600189, 16.26393749999999727, -2.595505584112000275 ) ) ;
#8416=CARTESIAN_POINT ( 'NONE',  ( 12.88040283537677588, 12.29391749999999739, -0.09070320285213756550 ) ) ;
#8442=AXIS2_PLACEMENT_3D ( 'NONE', #9529, #9197, #5885 ) ;
#8486=DIRECTION ( 'NONE',  ( 0.000000000000000000, 1.000000000000000000, 0.000000000000000000 ) ) ;
#8515=VECTOR ( 'NONE', #11059, 1000.000000000000000 ) ;
#8519=CARTESIAN_POINT ( 'NONE',  ( 31.06384331886062711, 2.019535839764540430, 1.146004012482531476 ) ) ;
#8594=DIRECTION ( 'NONE',  ( -0.9579671649362032637, 0.000000000000000000, 0.2868778675745010664 ) ) ;
#8597=EDGE_LOOP ( 'NONE', ( #8374, #2408, #8599, #7350, #12565, #20201, #4958, #891, #21710, #17751, #6230, #18622, #6260, #13138, #11604, #1586, #15759, #10248, #5488, #980, #1991, #9121 ) ) ;
#8598=EDGE_CURVE ( 'NONE', #4584, #4404, #17016, .T. ) ;
#8599=ORIENTED_EDGE ( 'NONE', *, *, #5742, .T. ) ;
#8602=DIRECTION ( 'NONE',  ( 0.2868778675745011220, 0.000000000000000000, 0.9579671649362034858 ) ) ;
#8604=ORIENTED_EDGE ( 'NONE', *, *, #11830, .T. ) ;
#8676=CARTESIAN_POINT ( 'NONE',  ( 30.02465935949302533, 2.019535839764540430, -2.324128137548288731 ) ) ;
#8677=DIRECTION ( 'NONE',  ( -0.2868778675745011220, 0.000000000000000000, -0.9579671649362034858 ) ) ;
#8720=DIRECTION ( 'NONE',  ( 0.2868778675745011220, 0.000000000000000000, 0.9579671649362034858 ) ) ;
#8733=CARTESIAN_POINT ( 'NONE',  ( 12.88040283537677588, 13.08893749999999834, -0.09070320285213756550 ) ) ;
#8756=ORIENTED_EDGE ( 'NONE', *, *, #6925, .F. ) ;
#8772=FACE_OUTER_BOUND ( 'NONE', #12318, .T. ) ;
#8843=ORIENTED_EDGE ( 'NONE', *, *, #17042, .F. ) ;
#8886=VECTOR ( 'NONE', #6396, 1000.000000000000000 ) ;
#8888=CARTESIAN_POINT ( 'NONE',  ( 30.78626241496060700, 0.001587500000000546807, -2.552201779827368622 ) ) ;
#8907=VECTOR ( 'NONE', #20620, 1000.000000000000227 ) ;
#8913=DIRECTION ( 'NONE',  ( 0.2868778675745011220, 0.000000000000000000, 0.9579671649362033747 ) ) ;
#8960=CARTESIAN_POINT ( 'NONE',  ( 24.71252020198295085, 23.75961143032650114, -0.7333271064221494884 ) ) ;
#8968=EDGE_CURVE ( 'NONE', #1968, #20661, #9578, .T. ) ;
#8988=FILL_AREA_STYLE_COLOUR ( '', #19454 ) ;
#8991=CIRCLE ( 'NONE', #16437, 0.7950200000000003930 ) ;
#9013=ORIENTED_EDGE ( 'NONE', *, *, #544, .T. ) ;
#9015=CARTESIAN_POINT ( 'NONE',  ( 1.854799496439154316, 13.08893749999999834, 3.211081754263136911 ) ) ;
#9028=CARTESIAN_POINT ( 'NONE',  ( 13.67756757867809725, 12.29391749999999739, 2.571257636385987144 ) ) ;
#9029=DIRECTION ( 'NONE',  ( -0.9564948366894091558, 0.05542109139015080621, 0.2864369564417710845 ) ) ;
#9058=DIRECTION ( 'NONE',  ( 0.2868778675745011220, 0.000000000000000000, 0.9579671649362034858 ) ) ;
#9063=CYLINDRICAL_SURFACE ( 'NONE', #12374, 0.7950199999999996159 ) ;
#9096=ADVANCED_FACE ( 'NONE', ( #3291 ), #1616, .T. ) ;
#9113=DIRECTION ( 'NONE',  ( 0.9579671649362032637, 0.000000000000000000, -0.2868778675745010664 ) ) ;
#9121=ORIENTED_EDGE ( 'NONE', *, *, #16069, .F. ) ;
#9143=EDGE_CURVE ( 'NONE', #10936, #20661, #7148, .T. ) ;
#9197=DIRECTION ( 'NONE',  ( 0.2868778675745011220, 0.000000000000000000, 0.9579671649362034858 ) ) ;
#9221=EDGE_CURVE ( 'NONE', #13909, #18557, #11796, .T. ) ;
#9231=CLOSED_SHELL ( 'NONE', ( #21826, #12597, #6852, #3182, #3585, #12612, #20119, #10996, #19671, #6949, #17071, #9096, #13483, #4136, #6703, #14723, #10981, #10004, #6081, #21521, #6706, #2999, #453, #16679, #868, #19211, #9352, #20616 ) ) ;
#9264=DIRECTION ( 'NONE',  ( -0.2868778675745011220, 0.000000000000000000, -0.9579671649362034858 ) ) ;
#9268=EDGE_CURVE ( 'NONE', #17651, #21745, #12007, .T. ) ;
#9291=DIRECTION ( 'NONE',  ( 0.2868778675745011220, 0.000000000000000000, 0.9579671649362034858 ) ) ;
#9329=CARTESIAN_POINT ( 'NONE',  ( 12.11879977990919421, 12.29391749999999739, 0.1373704394269426865 ) ) ;
#9340=( LENGTH_UNIT ( ) NAMED_UNIT ( * ) SI_UNIT ( .MILLI., .METRE. ) );
#9352=ADVANCED_FACE ( 'NONE', ( #12570 ), #15896, .T. ) ;
#9354=AXIS2_PLACEMENT_3D ( 'NONE', #19870, #8044, #16145 ) ;
#9469=DIRECTION ( 'NONE',  ( 0.2868778675745010664, 0.000000000000000000, 0.9579671649362032637 ) ) ;
#9478=ORIENTED_EDGE ( 'NONE', *, *, #13978, .T. ) ;
#9479=AXIS2_PLACEMENT_3D ( 'NONE', #12796, #19619, #12909 ) ;
#9495=CARTESIAN_POINT ( 'NONE',  ( 12.88040283537677588, 38.48766750000000059, -0.09070320285213756550 ) ) ;
#9525=CIRCLE ( 'NONE', #17292, 3.175000000000000711 ) ;
#9529=CARTESIAN_POINT ( 'NONE',  ( 29.98909767165928386, 9.120187499999998337, -5.214162619065493054 ) ) ;
#9542=DIRECTION ( 'NONE',  ( 0.2868778675745011220, 0.000000000000000000, 0.9579671649362033747 ) ) ;
#9570=LINE ( 'NONE', #16341, #2244 ) ;
#9578=LINE ( 'NONE', #13257, #7802 ) ;
#9600=CARTESIAN_POINT ( 'NONE',  ( 13.64200589084435578, 38.48766750000000059, -0.3187768451312169571 ) ) ;
#9688=VERTEX_POINT ( 'NONE', #11773 ) ;
#9702=DIRECTION ( 'NONE',  ( 0.000000000000000000, 1.000000000000000000, 0.000000000000000000 ) ) ;
#9756=CARTESIAN_POINT ( 'NONE',  ( 24.43309469626978725, 23.18727947754285879, -0.6496488801123181389 ) ) ;
#9794=DIRECTION ( 'NONE',  ( 0.000000000000000000, -1.000000000000000000, 0.000000000000000000 ) ) ;
#9817=ORIENTED_EDGE ( 'NONE', *, *, #16520, .F. ) ;
#9821=ORIENTED_EDGE ( 'NONE', *, *, #9268, .T. ) ;
#9841=ORIENTED_EDGE ( 'NONE', *, *, #8390, .F. ) ;
#9845=DIRECTION ( 'NONE',  ( -0.2868778675745011220, 0.000000000000000000, -0.9579671649362034858 ) ) ;
#9853=DIRECTION ( 'NONE',  ( 0.9579671649362033747, 0.000000000000000000, -0.2868778675745006779 ) ) ;
#9906=AXIS2_PLACEMENT_3D ( 'NONE', #6700, #13915, #20494 ) ;
#9918=EDGE_CURVE ( 'NONE', #17422, #16118, #16860, .T. ) ;
#9941=CIRCLE ( 'NONE', #4652, 0.7950199999999990608 ) ;
#9944=EDGE_CURVE ( 'NONE', #10623, #15859, #8292, .T. ) ;
#9955=LINE ( 'NONE', #11733, #3614 ) ;
#9985=LINE ( 'NONE', #14770, #12401 ) ;
#10004=ADVANCED_FACE ( 'NONE', ( #15605 ), #1980, .F. ) ;
#10062=ORIENTED_EDGE ( 'NONE', *, *, #15494, .T. ) ;
#10079=CARTESIAN_POINT ( 'NONE',  ( 12.11879977990919421, 20.23395749999999893, 0.1373704394269426865 ) ) ;
#10112=FACE_OUTER_BOUND ( 'NONE', #13240, .T. ) ;
#10121=LINE ( 'NONE', #16867, #19129 ) ;
#10183=DIRECTION ( 'NONE',  ( 0.9579671649362032637, 0.000000000000000000, -0.2868778675745010664 ) ) ;
#10201=ORIENTED_EDGE ( 'NONE', *, *, #9143, .F. ) ;
#10207=( NAMED_UNIT ( * ) SI_UNIT ( $, .STERADIAN. ) SOLID_ANGLE_UNIT ( ) );
#10235=ORIENTED_EDGE ( 'NONE', *, *, #14170, .F. ) ;
#10244=DIRECTION ( 'NONE',  ( 0.2868778675745010664, 0.000000000000000000, 0.9579671649362032637 ) ) ;
#10248=ORIENTED_EDGE ( 'NONE', *, *, #11830, .F. ) ;
#10260=ORIENTED_EDGE ( 'NONE', *, *, #16069, .T. ) ;
#10282=CARTESIAN_POINT ( 'NONE',  ( 26.41404040124396602, 0.001587500000000546807, -1.242873262350622010 ) ) ;
#10312=CIRCLE ( 'NONE', #19479, 6.350000000000005862 ) ;
#10343=ORIENTED_EDGE ( 'NONE', *, *, #9268, .F. ) ;
#10361=AXIS2_PLACEMENT_3D ( 'NONE', #11070, #17826, #1401 ) ;
#10391=DIRECTION ( 'NONE',  ( -0.2868778675745010664, 0.000000000000000000, -0.9579671649362032637 ) ) ;
#10410=FACE_OUTER_BOUND ( 'NONE', #13168, .T. ) ;
#10456=DIRECTION ( 'NONE',  ( 0.2868778675745011220, 0.000000000000000000, 0.9579671649362034858 ) ) ;
#10460=DIRECTION ( 'NONE',  ( 0.9579671649362032637, 0.000000000000000000, -0.2868778675745010664 ) ) ;
#10474=CARTESIAN_POINT ( 'NONE',  ( 29.98909767165928386, 23.40768749999999798, -5.214162619065493054 ) ) ;
#10492=CARTESIAN_POINT ( 'NONE',  ( 29.98909767165928386, 30.50833916023545811, -5.214162619065493054 ) ) ;
#10539=( LENGTH_UNIT ( ) NAMED_UNIT ( * ) SI_UNIT ( .MILLI., .METRE. ) );
#10560=DIRECTION ( 'NONE',  ( 0.9579671649362033747, 0.000000000000000000, -0.2868778675745006779 ) ) ;
#10585=CARTESIAN_POINT ( 'NONE',  ( 24.71252020198295085, 8.768263569673496960, -0.7333271064221494884 ) ) ;
#10607=LINE ( 'NONE', #10492, #16676 ) ;
#10623=VERTEX_POINT ( 'NONE', #20671 ) ;
#10718=AXIS2_PLACEMENT_3D ( 'NONE', #12735, #9291, #19459 ) ;
#10736=DIRECTION ( 'NONE',  ( 0.2868778675745011220, 0.000000000000000000, 0.9579671649362034858 ) ) ;
#10760=EDGE_CURVE ( 'NONE', #20009, #18286, #19572, .T. ) ;
#10771=VECTOR ( 'NONE', #19621, 1000.000000000000227 ) ;
#10808=ORIENTED_EDGE ( 'NONE', *, *, #13339, .T. ) ;
#10810=DIRECTION ( 'NONE',  ( 0.000000000000000000, -1.000000000000000000, 0.000000000000000000 ) ) ;
#10829=PLANE ( 'NONE',  #7132 ) ;
#10837=PLANE ( 'NONE',  #20700 ) ;
#10865=ORIENTED_EDGE ( 'NONE', *, *, #8323, .T. ) ;
#10885=( GEOMETRIC_REPRESENTATION_CONTEXT ( 3 ) GLOBAL_UNCERTAINTY_ASSIGNED_CONTEXT ( ( #4144 ) ) GLOBAL_UNIT_ASSIGNED_CONTEXT ( ( #9340, #20254, #10207 ) ) REPRESENTATION_CONTEXT ( 'NONE', 'WORKASPACE' ) );
#10888=VERTEX_POINT ( 'NONE', #10896 ) ;
#10896=CARTESIAN_POINT ( 'NONE',  ( 23.91535545868163126, 8.768263569673496960, -3.395287945660274254 ) ) ;
#10936=VERTEX_POINT ( 'NONE', #12676 ) ;
#10980=EDGE_CURVE ( 'NONE', #7865, #17422, #16558, .T. ) ;
#10981=ADVANCED_FACE ( 'NONE', ( #21167 ), #6022, .T. ) ;
#10993=PRODUCT_DEFINITION_CONTEXT ( 'detailed design', #983, 'design' ) ;
#10996=ADVANCED_FACE ( 'NONE', ( #1049 ), #4487, .T. ) ;
#11010=ORIENTED_EDGE ( 'NONE', *, *, #8390, .T. ) ;
#11018=SHAPE_REPRESENTATION ( 'Frame Locking Pawl Plate', ( #2234 ), #10885 ) ;
#11044=FACE_OUTER_BOUND ( 'NONE', #11878, .T. ) ;
#11046=DIRECTION ( 'NONE',  ( -0.2868778675745011220, 0.000000000000000000, -0.9579671649362034858 ) ) ;
#11059=DIRECTION ( 'NONE',  ( 0.000000000000000000, 1.000000000000000000, 0.000000000000000000 ) ) ;
#11070=CARTESIAN_POINT ( 'NONE',  ( 15.47835459351327714, -5.959792500000001603, 5.813316144137728791 ) ) ;
#11117=ORIENTED_EDGE ( 'NONE', *, *, #15060, .F. ) ;
#11157=DIRECTION ( 'NONE',  ( 0.9564948366894089338, -0.05542109139015086172, -0.2864369564417716951 ) ) ;
#11181=ORIENTED_EDGE ( 'NONE', *, *, #14170, .T. ) ;
#11209=FACE_OUTER_BOUND ( 'NONE', #2752, .T. ) ;
#11248=PRODUCT_DEFINITION_FORMATION_WITH_SPECIFIED_SOURCE ( 'ANY', '', #6509, .NOT_KNOWN. ) ;
#11250=EDGE_LOOP ( 'NONE', ( #12932, #10260, #7577, #3644 ) ) ;
#11251=EDGE_CURVE ( 'NONE', #16568, #3519, #4186, .T. ) ;
#11277=CIRCLE ( 'NONE', #16921, 0.7950200000000010592 ) ;
#11324=ORIENTED_EDGE ( 'NONE', *, *, #15646, .T. ) ;
#11328=DIRECTION ( 'NONE',  ( 0.9579671649362032637, 0.000000000000000000, -0.2868778675745010664 ) ) ;
#11336=DIRECTION ( 'NONE',  ( 0.000000000000000000, -1.000000000000000000, -0.000000000000000000 ) ) ;
#11372=CARTESIAN_POINT ( 'NONE',  ( 30.78626241496060700, 9.120187499999998337, -2.552201779827368622 ) ) ;
#11377=VECTOR ( 'NONE', #5095, 1000.000000000000227 ) ;
#11424=CARTESIAN_POINT ( 'NONE',  ( 29.98909767165928386, -5.959792500000001603, -5.214162619065493054 ) ) ;
#11439=ORIENTED_EDGE ( 'NONE', *, *, #7960, .F. ) ;
#11458=DIRECTION ( 'NONE',  ( 0.9564948366894089338, -0.05542109139015086172, -0.2864369564417716951 ) ) ;
#11476=DIRECTION ( 'NONE',  ( -0.2868778675745010664, 0.000000000000000000, -0.9579671649362032637 ) ) ;
#11478=AXIS2_PLACEMENT_3D ( 'NONE', #4518, #12832, #16254 ) ;
#11521=VERTEX_POINT ( 'NONE', #15044 ) ;
#11559=DIRECTION ( 'NONE',  ( -0.2868778675745011220, 0.000000000000000000, -0.9579671649362034858 ) ) ;
#11587=FACE_OUTER_BOUND ( 'NONE', #20533, .T. ) ;
#11591=ORIENTED_EDGE ( 'NONE', *, *, #9221, .F. ) ;
#11604=ORIENTED_EDGE ( 'NONE', *, *, #4535, .T. ) ;
#11666=AXIS2_PLACEMENT_3D ( 'NONE', #18260, #1666, #18364 ) ;
#11689=ORIENTED_EDGE ( 'NONE', *, *, #11251, .F. ) ;
#11733=CARTESIAN_POINT ( 'NONE',  ( 13.67756757867809725, 12.29391749999999739, 2.571257636385987144 ) ) ;
#11747=DIRECTION ( 'NONE',  ( 0.000000000000000000, -1.000000000000000000, 0.000000000000000000 ) ) ;
#11773=CARTESIAN_POINT ( 'NONE',  ( 1.854799496439154316, 13.08893749999999834, 3.211081754263136911 ) ) ;
#11796=LINE ( 'NONE', #61, #6379 ) ;
#11830=EDGE_CURVE ( 'NONE', #7786, #13109, #20297, .T. ) ;
#11837=DIRECTION ( 'NONE',  ( -0.2868778675745010664, 0.000000000000000000, -0.9579671649362032637 ) ) ;
#11844=CARTESIAN_POINT ( 'NONE',  ( 29.22749461619170219, -5.959792500000001603, -4.986088976786413163 ) ) ;
#11853=CARTESIAN_POINT ( 'NONE',  ( 12.88040283537677588, 38.48766750000000059, -0.09070320285213756550 ) ) ;
#11878=EDGE_LOOP ( 'NONE', ( #20937, #21634, #21638, #9841, #13781, #3920 ) ) ;
#11880=EDGE_CURVE ( 'NONE', #11521, #21727, #4285, .T. ) ;
#11906=ORIENTED_EDGE ( 'NONE', *, *, #15494, .F. ) ;
#11998=CARTESIAN_POINT ( 'NONE',  ( 30.78626241496060700, 32.52628750000000224, -2.552201779827368622 ) ) ;
#12007=LINE ( 'NONE', #18738, #15553 ) ;
#12029=EDGE_LOOP ( 'NONE', ( #18222, #16718, #19009, #20087 ) ) ;
#12036=EDGE_LOOP ( 'NONE', ( #17607, #20144, #5099, #18158 ) ) ;
#12093=FACE_OUTER_BOUND ( 'NONE', #2182, .T. ) ;
#12116=UNCERTAINTY_MEASURE_WITH_UNIT (LENGTH_MEASURE( 1.000000000000000082E-05 ), #10539, 'distance_accuracy_value', 'NONE');
#12232=VERTEX_POINT ( 'NONE', #2707 ) ;
#12233=CARTESIAN_POINT ( 'NONE',  ( 30.78626241496060700, 38.48766750000000059, -2.552201779827368622 ) ) ;
#12241=AXIS2_PLACEMENT_3D ( 'NONE', #2324, #9058, #4432 ) ;
#12268=DIRECTION ( 'NONE',  ( 0.000000000000000000, 1.000000000000000000, 0.000000000000000000 ) ) ;
#12285=ORIENTED_EDGE ( 'NONE', *, *, #2073, .F. ) ;
#12300=CARTESIAN_POINT ( 'NONE',  ( 29.98909767165928386, 9.120187499999998337, -5.214162619065493054 ) ) ;
#12312=SHAPE_DEFINITION_REPRESENTATION ( #14096, #11018 ) ;
#12318=EDGE_LOOP ( 'NONE', ( #11689, #12285, #7207, #2254 ) ) ;
#12349=ORIENTED_EDGE ( 'NONE', *, *, #18262, .T. ) ;
#12358=VECTOR ( 'NONE', #21120, 1000.000000000000227 ) ;
#12374=AXIS2_PLACEMENT_3D ( 'NONE', #20555, #19011, #2329 ) ;
#12384=DIRECTION ( 'NONE',  ( 0.1065921516619544457, 0.9937903127262237568, -0.03192064434796771516 ) ) ;
#12401=VECTOR ( 'NONE', #16742, 1000.000000000000227 ) ;
#12419=DIRECTION ( 'NONE',  ( -0.2868778675745011220, 0.000000000000000000, -0.9579671649362034858 ) ) ;
#12431=FACE_OUTER_BOUND ( 'NONE', #20159, .T. ) ;
#12435=SURFACE_STYLE_FILL_AREA ( #2131 ) ;
#12450=EDGE_CURVE ( 'NONE', #13109, #9688, #4131, .T. ) ;
#12491=VECTOR ( 'NONE', #11476, 1000.000000000000227 ) ;
#12509=VERTEX_POINT ( 'NONE', #2875 ) ;
#12549=VERTEX_POINT ( 'NONE', #9495 ) ;
#12565=ORIENTED_EDGE ( 'NONE', *, *, #5849, .T. ) ;
#12570=FACE_OUTER_BOUND ( 'NONE', #3599, .T. ) ;
#12597=ADVANCED_FACE ( 'NONE', ( #16054 ), #10837, .T. ) ;
#12612=ADVANCED_FACE ( 'NONE', ( #15946 ), #6726, .T. ) ;
#12634=CARTESIAN_POINT ( 'NONE',  ( 22.04181838752732148, 16.26393749999999727, 0.06645525512612464325 ) ) ;
#12640=ORIENTED_EDGE ( 'NONE', *, *, #17426, .T. ) ;
#12641=LINE ( 'NONE', #2573, #3237 ) ;
#12676=CARTESIAN_POINT ( 'NONE',  ( 30.78626241496060700, 1.982787499999999481, -2.552201779827368622 ) ) ;
#12709=CARTESIAN_POINT ( 'NONE',  ( 13.67756757867809725, 38.48766750000000059, 2.571257636385987144 ) ) ;
#12735=CARTESIAN_POINT ( 'NONE',  ( 14.43917063414567536, -5.959792500000001603, 2.343183994106907697 ) ) ;
#12796=CARTESIAN_POINT ( 'NONE',  ( 24.99127163628573456, 8.724202693596797786, 2.964528152719008158 ) ) ;
#12814=CARTESIAN_POINT ( 'NONE',  ( 30.10940225190841701, 29.71825598581263961, -2.349505688218141319 ) ) ;
#12832=DIRECTION ( 'NONE',  ( 0.9579671649362033747, 0.000000000000000000, -0.2868778675745011220 ) ) ;
#12909=DIRECTION ( 'NONE',  ( 0.6050250551579474667, 0.7753173868113220069, -0.1811839737371539749 ) ) ;
#12929=ORIENTED_EDGE ( 'NONE', *, *, #13815, .T. ) ;
#12932=ORIENTED_EDGE ( 'NONE', *, *, #1883, .T. ) ;
#12944=EDGE_CURVE ( 'NONE', #13358, #20009, #3624, .T. ) ;
#12969=AXIS2_PLACEMENT_3D ( 'NONE', #21871, #18236, #14944 ) ;
#12983=CARTESIAN_POINT ( 'NONE',  ( 30.10940225190841701, 29.71825598581263961, -2.349505688218141319 ) ) ;
#12989=CARTESIAN_POINT ( 'NONE',  ( 23.95208767691813279, 23.80367230640320031, -0.5056039973118116038 ) ) ;
#13070=EDGE_CURVE ( 'NONE', #15859, #93, #4146, .T. ) ;
#13077=DIRECTION ( 'NONE',  ( 0.1065921516619546816, -0.9937903127262236458, -0.03192064434796833272 ) ) ;
#13096=AXIS2_PLACEMENT_3D ( 'NONE', #8733, #4438, #7633 ) ;
#13109=VERTEX_POINT ( 'NONE', #15911 ) ;
#13134=CARTESIAN_POINT ( 'NONE',  ( 29.31223750860709742, 2.809619014187358932, -5.011466527456265752 ) ) ;
#13138=ORIENTED_EDGE ( 'NONE', *, *, #4898, .F. ) ;
#13155=AXIS2_PLACEMENT_3D ( 'NONE', #5391, #8602, #8486 ) ;
#13168=EDGE_LOOP ( 'NONE', ( #4498, #21004, #19886, #14898, #7501, #7704 ) ) ;
#13174=CIRCLE ( 'NONE', #16696, 0.7950200000000010592 ) ;
#13188=VERTEX_POINT ( 'NONE', #13134 ) ;
#13213=CARTESIAN_POINT ( 'NONE',  ( 30.02465935949302533, 38.48766750000000059, -2.324128137548288731 ) ) ;
#13227=LINE ( 'NONE', #16431, #16593 ) ;
#13240=EDGE_LOOP ( 'NONE', ( #5019, #7832, #5515, #5555 ) ) ;
#13257=CARTESIAN_POINT ( 'NONE',  ( 13.67756757867809725, 12.29391749999999739, 2.571257636385987144 ) ) ;
#13339=EDGE_CURVE ( 'NONE', #21727, #21745, #13670, .T. ) ;
#13355=DIRECTION ( 'NONE',  ( -0.2868778675745011220, 0.000000000000000000, -0.9579671649362034858 ) ) ;
#13358=VERTEX_POINT ( 'NONE', #11998 ) ;
#13386=DIRECTION ( 'NONE',  ( 0.9579671649362032637, 0.000000000000000000, -0.2868778675745012885 ) ) ;
#13408=DIRECTION ( 'NONE',  ( 0.000000000000000000, -1.000000000000000000, 0.000000000000000000 ) ) ;
#13440=CARTESIAN_POINT ( 'NONE',  ( 30.78626241496060700, -5.959792500000001603, -2.552201779827368622 ) ) ;
#13465=VECTOR ( 'NONE', #1104, 1000.000000000000227 ) ;
#13483=ADVANCED_FACE ( 'NONE', ( #8772 ), #15552, .T. ) ;
#13496=VECTOR ( 'NONE', #5299, 1000.000000000000227 ) ;
#13593=CARTESIAN_POINT ( 'NONE',  ( 13.67756757867809725, 12.29391749999999739, 2.571257636385987144 ) ) ;
#13607=ORIENTED_EDGE ( 'NONE', *, *, #18883, .T. ) ;
#13622=CARTESIAN_POINT ( 'NONE',  ( 12.91596452321051558, 19.43893749999999798, 2.799331278665067479 ) ) ;
#13633=CYLINDRICAL_SURFACE ( 'NONE', #18365, 0.7950200000000003930 ) ;
#13637=DIRECTION ( 'NONE',  ( -0.9579671649362032637, -2.486588751566399063E-16, 0.2868778675745010664 ) ) ;
#13670=LINE ( 'NONE', #500, #357 ) ;
#13728=DIRECTION ( 'NONE',  ( -0.9579671649362032637, 0.000000000000000000, 0.2868778675745010664 ) ) ;
#13729=ORIENTED_EDGE ( 'NONE', *, *, #14952, .F. ) ;
#13737=CARTESIAN_POINT ( 'NONE',  ( 23.91535545868163126, 23.75961143032650114, -3.395287945660274254 ) ) ;
#13750=CARTESIAN_POINT ( 'NONE',  ( 13.67756757867809725, 30.54508749999999750, 2.571257636385987144 ) ) ;
#13781=ORIENTED_EDGE ( 'NONE', *, *, #19723, .T. ) ;
#13805=CARTESIAN_POINT ( 'NONE',  ( 30.78626241496060700, 30.50833916023545811, -2.552201779827368622 ) ) ;
#13815=EDGE_CURVE ( 'NONE', #699, #1968, #9985, .T. ) ;
#13830=AXIS2_PLACEMENT_3D ( 'NONE', #21164, #7359, #9113 ) ;
#13838=DIRECTION ( 'NONE',  ( 0.2868778675745011220, 0.000000000000000000, 0.9579671649362033747 ) ) ;
#13870=CARTESIAN_POINT ( 'NONE',  ( 11.07961582054159244, 20.23395749999999893, -3.332761710603877159 ) ) ;
#13906=DIRECTION ( 'NONE',  ( 0.9579671649362033747, 0.000000000000000000, -0.2868778675745006779 ) ) ;
#13909=VERTEX_POINT ( 'NONE', #5437 ) ;
#13915=DIRECTION ( 'NONE',  ( 0.000000000000000000, -1.000000000000000000, -0.000000000000000000 ) ) ;
#13935=AXIS2_PLACEMENT_3D ( 'NONE', #16359, #21529, #9702 ) ;
#13970=ORIENTED_EDGE ( 'NONE', *, *, #19779, .T. ) ;
#13978=EDGE_CURVE ( 'NONE', #20529, #4584, #1678, .T. ) ;
#13999=PRESENTATION_STYLE_ASSIGNMENT (( #2471 ) ) ;
#14022=CARTESIAN_POINT ( 'NONE',  ( 0.000000000000000000, 0.000000000000000000, 0.000000000000000000 ) ) ;
#14060=EDGE_LOOP ( 'NONE', ( #8077, #18414, #19862, #21378 ) ) ;
#14073=LINE ( 'NONE', #20433, #2834 ) ;
#14093=DIRECTION ( 'NONE',  ( -0.2868778675745010664, 0.000000000000000000, -0.9579671649362032637 ) ) ;
#14096=PRODUCT_DEFINITION_SHAPE ( 'NONE', 'NONE',  #17378 ) ;
#14165=DIRECTION ( 'NONE',  ( 0.000000000000000000, 1.000000000000000000, 0.000000000000000000 ) ) ;
#14170=EDGE_CURVE ( 'NONE', #18658, #3169, #12641, .T. ) ;
#14181=DIRECTION ( 'NONE',  ( 0.9579671649362032637, 0.000000000000000000, -0.2868778675745010664 ) ) ;
#14182=CARTESIAN_POINT ( 'NONE',  ( 23.95208767691813279, 8.724202693596797786, -0.5056039973118116038 ) ) ;
#14217=DIRECTION ( 'NONE',  ( -0.2868778675745010664, 0.000000000000000000, -0.9579671649362032637 ) ) ;
#14226=VECTOR ( 'NONE', #8051, 1000.000000000000000 ) ;
#14338=ADVANCED_BREP_SHAPE_REPRESENTATION ( '', ( #6428, #2234 ), #10885 ) ;
#14358=DIRECTION ( 'NONE',  ( -0.2868778675745010664, 0.000000000000000000, -0.9579671649362032637 ) ) ;
#14421=VECTOR ( 'NONE', #11837, 1000.000000000000227 ) ;
#14450=DIRECTION ( 'NONE',  ( -0.9564948366894091558, 0.05542109139015083397, 0.2864369564417712510 ) ) ;
#14456=ORIENTED_EDGE ( 'NONE', *, *, #17647, .T. ) ;
#14509=VECTOR ( 'NONE', #11747, 1000.000000000000000 ) ;
#14559=DIRECTION ( 'NONE',  ( 0.2868778675745010664, 0.000000000000000000, 0.9579671649362032637 ) ) ;
#14600=AXIS2_PLACEMENT_3D ( 'NONE', #2075, #17233, #13386 ) ;
#14602=VECTOR ( 'NONE', #4470, 1000.000000000000000 ) ;
#14606=FACE_OUTER_BOUND ( 'NONE', #21829, .T. ) ;
#14642=EDGE_LOOP ( 'NONE', ( #8017, #20766, #1191, #2416 ) ) ;
#14649=LINE ( 'NONE', #12983, #21500 ) ;
#14665=DIRECTION ( 'NONE',  ( 0.9579671649362032637, 0.000000000000000000, -0.2868778675745010664 ) ) ;
#14700=ORIENTED_EDGE ( 'NONE', *, *, #1115, .T. ) ;
#14711=DIRECTION ( 'NONE',  ( -0.2868778675745011220, 0.000000000000000000, -0.9579671649362034858 ) ) ;
#14723=ADVANCED_FACE ( 'NONE', ( #12431 ), #2793, .F. ) ;
#14728=VERTEX_POINT ( 'NONE', #7557 ) ;
#14743=CARTESIAN_POINT ( 'NONE',  ( 30.02465935949302533, -5.959792500000001603, -2.324128137548288731 ) ) ;
#14765=CYLINDRICAL_SURFACE ( 'NONE', #17777, 6.350000000000001421 ) ;
#14770=CARTESIAN_POINT ( 'NONE',  ( 12.88040283537677588, 12.29391749999999739, -0.09070320285213756550 ) ) ;
#14802=ORIENTED_EDGE ( 'NONE', *, *, #21548, .T. ) ;
#14812=ORIENTED_EDGE ( 'NONE', *, *, #17598, .F. ) ;
#14814=VECTOR ( 'NONE', #10810, 1000.000000000000000 ) ;
#14898=ORIENTED_EDGE ( 'NONE', *, *, #8968, .F. ) ;
#14917=ORIENTED_EDGE ( 'NONE', *, *, #18010, .T. ) ;
#14938=DIRECTION ( 'NONE',  ( 0.2868778675745011220, 0.000000000000000000, 0.9579671649362034858 ) ) ;
#14944=DIRECTION ( 'NONE',  ( 0.9579671649362032637, 0.000000000000000000, -0.2868778675745010664 ) ) ;
#14952=EDGE_CURVE ( 'NONE', #17422, #4597, #14649, .T. ) ;
#15035=CIRCLE ( 'NONE', #9354, 0.7950200000000005041 ) ;
#15044=CARTESIAN_POINT ( 'NONE',  ( 13.67756757867809725, 32.52628750000000224, 2.571257636385987144 ) ) ;
#15060=EDGE_CURVE ( 'NONE', #12232, #21727, #3353, .T. ) ;
#15064=CARTESIAN_POINT ( 'NONE',  ( 24.43309469626978725, 9.340595522457139310, -0.6496488801123181389 ) ) ;
#15082=CARTESIAN_POINT ( 'NONE',  ( 26.41404040124396602, 30.54508749999999750, -1.242873262350622010 ) ) ;
#15176=CIRCLE ( 'NONE', #5676, 0.7950200000000005041 ) ;
#15195=DIRECTION ( 'NONE',  ( -0.9579671649362032637, 0.000000000000000000, 0.2868778675745010664 ) ) ;
#15230=CARTESIAN_POINT ( 'NONE',  ( 17.85969298310271114, 1.982787499999999481, 1.318856445756055873 ) ) ;
#15299=DIRECTION ( 'NONE',  ( 0.1065921516619544457, 0.9937903127262237568, -0.03192064434796798578 ) ) ;
#15304=CARTESIAN_POINT ( 'NONE',  ( 2.651964239740473683, 16.26393749999999727, 5.873042593501262232 ) ) ;
#15312=CARTESIAN_POINT ( 'NONE',  ( 30.02465935949302533, 39.28268749999999443, -2.324128137548288731 ) ) ;
#15354=CARTESIAN_POINT ( 'NONE',  ( 13.64200589084435578, -6.754812500000002551, -0.3187768451312169571 ) ) ;
#15391=EDGE_CURVE ( 'NONE', #21133, #539, #9525, .T. ) ;
#15398=AXIS2_PLACEMENT_3D ( 'NONE', #9329, #3842, #3734 ) ;
#15407=LINE ( 'NONE', #8960, #8123 ) ;
#15412=DIRECTION ( 'NONE',  ( 0.2868778675745011220, 0.000000000000000000, 0.9579671649362033747 ) ) ;
#15419=CARTESIAN_POINT ( 'NONE',  ( 30.02465935949302533, -6.754812500000002551, -2.324128137548288731 ) ) ;
#15451=DIRECTION ( 'NONE',  ( -0.6050250551579474667, -0.7753173868113220069, 0.1811839737371539194 ) ) ;
#15483=ORIENTED_EDGE ( 'NONE', *, *, #20741, .T. ) ;
#15494=EDGE_CURVE ( 'NONE', #11521, #13358, #17390, .T. ) ;
#15529=CYLINDRICAL_SURFACE ( 'NONE', #6448, 3.174999999999999822 ) ;
#15552=CYLINDRICAL_SURFACE ( 'NONE', #8116, 0.7950200000000010592 ) ;
#15553=VECTOR ( 'NONE', #14559, 1000.000000000000227 ) ;
#15602=LINE ( 'NONE', #2309, #503 ) ;
#15605=FACE_OUTER_BOUND ( 'NONE', #12029, .T. ) ;
#15613=ORIENTED_EDGE ( 'NONE', *, *, #9918, .F. ) ;
#15646=EDGE_CURVE ( 'NONE', #19832, #10888, #20313, .T. ) ;
#15682=ORIENTED_EDGE ( 'NONE', *, *, #7042, .T. ) ;
#15710=ORIENTED_EDGE ( 'NONE', *, *, #16168, .F. ) ;
#15725=AXIS2_PLACEMENT_3D ( 'NONE', #12989, #7666, #2695 ) ;
#15747=DIRECTION ( 'NONE',  ( 0.9579671649362032637, 1.243294375783199532E-16, -0.2868778675745010664 ) ) ;
#15750=EDGE_CURVE ( 'NONE', #4584, #304, #15602, .T. ) ;
#15754=DIRECTION ( 'NONE',  ( -0.1065921516619563053, -0.9937903127262235348, 0.03192064434796804129 ) ) ;
#15759=ORIENTED_EDGE ( 'NONE', *, *, #12450, .F. ) ;
#15798=CARTESIAN_POINT ( 'NONE',  ( 22.04181838752732148, 16.26393749999999727, 0.06645525512612464325 ) ) ;
#15838=DIRECTION ( 'NONE',  ( -0.2868778675745010664, 0.000000000000000000, -0.9579671649362032637 ) ) ;
#15859=VERTEX_POINT ( 'NONE', #21419 ) ;
#15896=PLANE ( 'NONE',  #13830 ) ;
#15911=CARTESIAN_POINT ( 'NONE',  ( 1.854799496439154316, 19.43893749999999798, 3.211081754263136911 ) ) ;
#15912=VERTEX_POINT ( 'NONE', #21313 ) ;
#15932=FACE_OUTER_BOUND ( 'NONE', #7564, .T. ) ;
#15946=FACE_OUTER_BOUND ( 'NONE', #2941, .T. ) ;
#15950=VERTEX_POINT ( 'NONE', #7589 ) ;
#15973=VECTOR ( 'NONE', #16497, 1000.000000000000227 ) ;
#15984=SURFACE_SIDE_STYLE ('',( #12435 ) ) ;
#15986=CIRCLE ( 'NONE', #1483, 0.7950200000000003930 ) ;
#16054=FACE_OUTER_BOUND ( 'NONE', #11250, .T. ) ;
#16065=AXIS2_PLACEMENT_3D ( 'NONE', #8152, #5353, #21646 ) ;
#16067=LINE ( 'NONE', #996, #12491 ) ;
#16069=EDGE_CURVE ( 'NONE', #15912, #304, #6244, .T. ) ;
#16112=CARTESIAN_POINT ( 'NONE',  ( 30.78626241496060700, 23.40768749999999798, -2.552201779827368622 ) ) ;
#16118=VERTEX_POINT ( 'NONE', #1165 ) ;
#16121=APPLICATION_CONTEXT ( 'automotive_design' ) ;
#16145=DIRECTION ( 'NONE',  ( 0.000000000000000000, -1.000000000000000000, 0.000000000000000000 ) ) ;
#16149=CARTESIAN_POINT ( 'NONE',  ( 12.88040283537677588, -5.959792500000001603, -0.09070320285213756550 ) ) ;
#16168=EDGE_CURVE ( 'NONE', #3169, #10936, #8339, .T. ) ;
#16235=ORIENTED_EDGE ( 'NONE', *, *, #6519, .F. ) ;
#16254=DIRECTION ( 'NONE',  ( 0.000000000000000000, 1.000000000000000000, 0.000000000000000000 ) ) ;
#16266=CIRCLE ( 'NONE', #21191, 0.7950200000000005041 ) ;
#16295=CARTESIAN_POINT ( 'NONE',  ( 13.64200589084435578, 39.28268749999999443, -0.3187768451312169571 ) ) ;
#16299=VECTOR ( 'NONE', #2037, 1000.000000000000227 ) ;
#16341=CARTESIAN_POINT ( 'NONE',  ( 30.78626241496060700, -5.959792500000001603, -2.552201779827368622 ) ) ;
#16342=CARTESIAN_POINT ( 'NONE',  ( 12.11879977990919421, 19.43893749999999798, 0.1373704394269426865 ) ) ;
#16359=CARTESIAN_POINT ( 'NONE',  ( 29.98909767165928386, 29.75768749999999940, -5.214162619065493054 ) ) ;
#16366=CARTESIAN_POINT ( 'NONE',  ( 29.22749461619170219, 30.50833916023545811, -4.986088976786413163 ) ) ;
#16413=EDGE_CURVE ( 'NONE', #4759, #7865, #17104, .T. ) ;
#16431=CARTESIAN_POINT ( 'NONE',  ( 14.43917063414567536, -6.754812500000002551, 2.343183994106907697 ) ) ;
#16437=AXIS2_PLACEMENT_3D ( 'NONE', #4627, #11046, #19755 ) ;
#16440=ORIENTED_EDGE ( 'NONE', *, *, #18429, .F. ) ;
#16463=ORIENTED_EDGE ( 'NONE', *, *, #4535, .F. ) ;
#16497=DIRECTION ( 'NONE',  ( 0.9579671649362032637, 0.000000000000000000, -0.2868778675745010664 ) ) ;
#16510=AXIS2_PLACEMENT_3D ( 'NONE', #2623, #17982, #17776 ) ;
#16520=EDGE_CURVE ( 'NONE', #7786, #21204, #1024, .T. ) ;
#16532=LINE ( 'NONE', #19938, #19518 ) ;
#16558=CIRCLE ( 'NONE', #1696, 6.350000000000002309 ) ;
#16568=VERTEX_POINT ( 'NONE', #11424 ) ;
#16581=CYLINDRICAL_SURFACE ( 'NONE', #7830, 0.7950199999999993938 ) ;
#16582=CARTESIAN_POINT ( 'NONE',  ( 23.15492293361681320, 23.80367230640320031, -3.167564836549936480 ) ) ;
#16584=ORIENTED_EDGE ( 'NONE', *, *, #8598, .T. ) ;
#16593=VECTOR ( 'NONE', #4810, 1000.000000000000227 ) ;
#16615=CYLINDRICAL_SURFACE ( 'NONE', #11666, 0.7950200000000010592 ) ;
#16621=CARTESIAN_POINT ( 'NONE',  ( 29.98909767165928386, 23.40768749999999798, -5.214162619065493054 ) ) ;
#16642=VECTOR ( 'NONE', #14217, 1000.000000000000227 ) ;
#16676=VECTOR ( 'NONE', #12268, 1000.000000000000000 ) ;
#16679=ADVANCED_FACE ( 'NONE', ( #3449 ), #3351, .F. ) ;
#16696=AXIS2_PLACEMENT_3D ( 'NONE', #13213, #16737, #9853 ) ;
#16718=ORIENTED_EDGE ( 'NONE', *, *, #13070, .T. ) ;
#16737=DIRECTION ( 'NONE',  ( 0.2868778675745011220, 0.000000000000000000, 0.9579671649362034858 ) ) ;
#16742=DIRECTION ( 'NONE',  ( 0.2868778675745010664, 0.000000000000000000, 0.9579671649362032637 ) ) ;
#16744=CARTESIAN_POINT ( 'NONE',  ( 1.854799496439154316, 16.26393749999999727, 3.211081754263136911 ) ) ;
#16860=CIRCLE ( 'NONE', #2751, 0.7950199999999986167 ) ;
#16863=CARTESIAN_POINT ( 'NONE',  ( 31.06384331886062711, -5.959792500000001603, 1.146004012482531476 ) ) ;
#16867=CARTESIAN_POINT ( 'NONE',  ( 1.854799496439154316, 13.08893749999999834, 3.211081754263136911 ) ) ;
#16921=AXIS2_PLACEMENT_3D ( 'NONE', #8676, #10456, #10560 ) ;
#16925=FACE_OUTER_BOUND ( 'NONE', #14060, .T. ) ;
#17016=CIRCLE ( 'NONE', #13155, 0.7950200000000005041 ) ;
#17029=AXIS2_PLACEMENT_3D ( 'NONE', #15798, #8913, #3951 ) ;
#17042=EDGE_CURVE ( 'NONE', #367, #13909, #6822, .T. ) ;
#17046=DIRECTION ( 'NONE',  ( 0.000000000000000000, 1.000000000000000000, 0.000000000000000000 ) ) ;
#17071=ADVANCED_FACE ( 'NONE', ( #19864 ), #4738, .T. ) ;
#17087=EDGE_CURVE ( 'NONE', #4759, #93, #16067, .T. ) ;
#17104=CIRCLE ( 'NONE', #15725, 0.7950199999999990608 ) ;
#17126=VERTEX_POINT ( 'NONE', #15354 ) ;
#17130=ORIENTED_EDGE ( 'NONE', *, *, #19607, .T. ) ;
#17132=CARTESIAN_POINT ( 'NONE',  ( 30.02465935949302533, 39.28268749999999443, -2.324128137548288731 ) ) ;
#17141=DIRECTION ( 'NONE',  ( 0.9579671649362032637, 0.000000000000000000, -0.2868778675745010664 ) ) ;
#17152=PLANE ( 'NONE',  #13096 ) ;
#17177=( NAMED_UNIT ( * ) PLANE_ANGLE_UNIT ( ) SI_UNIT ( $, .RADIAN. ) );
#17233=DIRECTION ( 'NONE',  ( -0.2868778675745011220, 0.000000000000000000, -0.9579671649362034858 ) ) ;
#17273=LINE ( 'NONE', #8416, #20305 ) ;
#17292=AXIS2_PLACEMENT_3D ( 'NONE', #15304, #18915, #17046 ) ;
#17356=CARTESIAN_POINT ( 'NONE',  ( 29.22749461619170219, 2.019535839764540430, -4.986088976786413163 ) ) ;
#17378=PRODUCT_DEFINITION ( 'UNKNOWN', '', #11248, #10993 ) ;
#17390=LINE ( 'NONE', #2230, #18499 ) ;
#17396=CARTESIAN_POINT ( 'NONE',  ( 30.78626241496060700, -5.959792500000001603, -2.552201779827368622 ) ) ;
#17422=VERTEX_POINT ( 'NONE', #12814 ) ;
#17425=ORIENTED_EDGE ( 'NONE', *, *, #18599, .T. ) ;
#17426=EDGE_CURVE ( 'NONE', #13109, #21133, #2843, .T. ) ;
#17471=FACE_OUTER_BOUND ( 'NONE', #18842, .T. ) ;
#17573=LINE ( 'NONE', #12709, #21698 ) ;
#17588=ORIENTED_EDGE ( 'NONE', *, *, #20797, .T. ) ;
#17598=EDGE_CURVE ( 'NONE', #15912, #18286, #15176, .T. ) ;
#17607=ORIENTED_EDGE ( 'NONE', *, *, #18429, .T. ) ;
#17644=DIRECTION ( 'NONE',  ( 1.000000000000000000, 0.000000000000000000, 0.000000000000000000 ) ) ;
#17647=EDGE_CURVE ( 'NONE', #5639, #12509, #11277, .T. ) ;
#17651=VERTEX_POINT ( 'NONE', #4046 ) ;
#17701=CARTESIAN_POINT ( 'NONE',  ( 2.651964239740473683, 13.08893749999999834, 5.873042593501262232 ) ) ;
#17751=ORIENTED_EDGE ( 'NONE', *, *, #21548, .F. ) ;
#17776=DIRECTION ( 'NONE',  ( -0.6050250551579474667, -0.7753173868113220069, 0.1811839737371539472 ) ) ;
#17777=AXIS2_PLACEMENT_3D ( 'NONE', #16621, #1348, #6117 ) ;
#17819=LINE ( 'NONE', #17701, #13465 ) ;
#17826=DIRECTION ( 'NONE',  ( -0.2868778675745011220, 0.000000000000000000, -0.9579671649362034858 ) ) ;
#17982=DIRECTION ( 'NONE',  ( -0.2868778675745011220, 0.000000000000000000, -0.9579671649362034858 ) ) ;
#18000=DIRECTION ( 'NONE',  ( 0.000000000000000000, 1.000000000000000000, 0.000000000000000000 ) ) ;
#18010=EDGE_CURVE ( 'NONE', #13909, #17126, #13227, .T. ) ;
#18025=AXIS2_PLACEMENT_3D ( 'NONE', #12300, #12419, #15754 ) ;
#18046=ORIENTED_EDGE ( 'NONE', *, *, #17426, .F. ) ;
#18068=CARTESIAN_POINT ( 'NONE',  ( 22.04181838752732148, 16.26393749999999727, 0.06645525512612464325 ) ) ;
#18127=DIRECTION ( 'NONE',  ( -0.9579671649362032637, 0.000000000000000000, 0.2868778675745013440 ) ) ;
#18158=ORIENTED_EDGE ( 'NONE', *, *, #5324, .T. ) ;
#18222=ORIENTED_EDGE ( 'NONE', *, *, #9944, .T. ) ;
#18236=DIRECTION ( 'NONE',  ( 0.000000000000000000, 1.000000000000000000, 0.000000000000000000 ) ) ;
#18251=DIRECTION ( 'NONE',  ( -0.2868778675745011220, 0.000000000000000000, -0.9579671649362034858 ) ) ;
#18260=CARTESIAN_POINT ( 'NONE',  ( 31.06384331886062711, 30.50833916023545811, 1.146004012482531476 ) ) ;
#18262=EDGE_CURVE ( 'NONE', #12509, #13188, #4543, .T. ) ;
#18286=VERTEX_POINT ( 'NONE', #2888 ) ;
#18287=SHAPE_REPRESENTATION_RELATIONSHIP ( 'NONE' , 'NONE' ,  #11018, #14338 ) ;
#18332=ORIENTED_EDGE ( 'NONE', *, *, #16520, .T. ) ;
#18352=LINE ( 'NONE', #2895, #15973 ) ;
#18364=DIRECTION ( 'NONE',  ( 0.9579671649362033747, 0.000000000000000000, -0.2868778675745006779 ) ) ;
#18365=AXIS2_PLACEMENT_3D ( 'NONE', #8519, #9845, #15299 ) ;
#18402=AXIS2_PLACEMENT_3D ( 'NONE', #14743, #6306, #4774 ) ;
#18414=ORIENTED_EDGE ( 'NONE', *, *, #18262, .F. ) ;
#18426=VECTOR ( 'NONE', #13728, 1000.000000000000227 ) ;
#18429=EDGE_CURVE ( 'NONE', #15950, #7495, #5485, .T. ) ;
#18434=CARTESIAN_POINT ( 'NONE',  ( 13.67756757867809725, 38.48766750000000059, 2.571257636385987144 ) ) ;
#18438=VERTEX_POINT ( 'NONE', #292 ) ;
#18487=FACE_OUTER_BOUND ( 'NONE', #2314, .T. ) ;
#18499=VECTOR ( 'NONE', #15747, 1000.000000000000227 ) ;
#18530=ORIENTED_EDGE ( 'NONE', *, *, #1883, .F. ) ;
#18545=FACE_OUTER_BOUND ( 'NONE', #19442, .T. ) ;
#18557=VERTEX_POINT ( 'NONE', #15419 ) ;
#18599=EDGE_CURVE ( 'NONE', #13188, #10888, #21180, .T. ) ;
#18611=ORIENTED_EDGE ( 'NONE', *, *, #20772, .F. ) ;
#18622=ORIENTED_EDGE ( 'NONE', *, *, #20179, .F. ) ;
#18658=VERTEX_POINT ( 'NONE', #17396 ) ;
#18738=CARTESIAN_POINT ( 'NONE',  ( 12.88040283537677588, 20.23395749999999893, -0.09070320285213756550 ) ) ;
#18829=AXIS2_PLACEMENT_3D ( 'NONE', #8405, #15412, #10183 ) ;
#18842=EDGE_LOOP ( 'NONE', ( #10201, #6106, #14456, #6599, #1157, #1317, #4772, #1504, #4753, #11010, #3656, #10808, #3511, #3618, #7262, #15682, #9013, #7738 ) ) ;
#18883=EDGE_CURVE ( 'NONE', #18557, #18658, #3900, .T. ) ;
#18906=DIRECTION ( 'NONE',  ( 0.000000000000000000, 1.000000000000000000, 0.000000000000000000 ) ) ;
#18915=DIRECTION ( 'NONE',  ( 0.2868778675745011220, 0.000000000000000000, 0.9579671649362034858 ) ) ;
#18919=DIRECTION ( 'NONE',  ( 0.2868778675745011220, 0.000000000000000000, 0.9579671649362034858 ) ) ;
#18966=FACE_OUTER_BOUND ( 'NONE', #2602, .T. ) ;
#19009=ORIENTED_EDGE ( 'NONE', *, *, #17087, .F. ) ;
#19011=DIRECTION ( 'NONE',  ( -0.2868778675745011220, 0.000000000000000000, -0.9579671649362034858 ) ) ;
#19041=CARTESIAN_POINT ( 'NONE',  ( 30.02465935949302533, -6.754812500000002551, -2.324128137548288731 ) ) ;
#19107=CARTESIAN_POINT ( 'NONE',  ( 31.06384331886062711, 38.48766750000000059, 1.146004012482531476 ) ) ;
#19117=CARTESIAN_POINT ( 'NONE',  ( 30.78626241496060700, 2.019535839764540430, -2.552201779827368622 ) ) ;
#19129=VECTOR ( 'NONE', #5546, 1000.000000000000227 ) ;
#19153=LINE ( 'NONE', #5039, #19456 ) ;
#19156=CARTESIAN_POINT ( 'NONE',  ( 23.63592995296846766, 23.18727947754285879, -3.311609719350443015 ) ) ;
#19186=CARTESIAN_POINT ( 'NONE',  ( 12.91596452321051558, 13.08893749999999834, 2.799331278665067479 ) ) ;
#19211=ADVANCED_FACE ( 'NONE', ( #17471 ), #10829, .T. ) ;
#19401=EDGE_CURVE ( 'NONE', #12232, #13358, #19556, .T. ) ;
#19423=VERTEX_POINT ( 'NONE', #16149 ) ;
#19442=EDGE_LOOP ( 'NONE', ( #12929, #6588, #16440, #16463 ) ) ;
#19445=CARTESIAN_POINT ( 'NONE',  ( 30.78626241496060700, 30.50833916023545811, -2.552201779827368622 ) ) ;
#19454=COLOUR_RGB ( '', 0.31764706, 0.68627451, 0.89019608) ;
#19456=VECTOR ( 'NONE', #14093, 1000.000000000000227 ) ;
#19459=DIRECTION ( 'NONE',  ( -0.9579671649362032637, 0.000000000000000000, 0.2868778675745012885 ) ) ;
#19479=AXIS2_PLACEMENT_3D ( 'NONE', #10474, #20629, #9029 ) ;
#19518=VECTOR ( 'NONE', #11328, 1000.000000000000227 ) ;
#19556=LINE ( 'NONE', #2754, #14226 ) ;
#19557=DIRECTION ( 'NONE',  ( -0.2868778675745011220, 0.000000000000000000, -0.9579671649362034858 ) ) ;
#19572=LINE ( 'NONE', #12233, #2041 ) ;
#19574=AXIS2_PLACEMENT_3D ( 'NONE', #11372, #9264, #4305 ) ;
#19602=CARTESIAN_POINT ( 'NONE',  ( 29.98909767165928386, -5.959792500000001603, -5.214162619065493054 ) ) ;
#19604=CARTESIAN_POINT ( 'NONE',  ( 29.31223750860709742, 29.71825598581263961, -5.011466527456265752 ) ) ;
#19607=EDGE_CURVE ( 'NONE', #1499, #367, #6610, .T. ) ;
#19619=DIRECTION ( 'NONE',  ( -0.2868778675745011220, 0.000000000000000000, -0.9579671649362034858 ) ) ;
#19621=DIRECTION ( 'NONE',  ( -0.9579671649362032637, 0.000000000000000000, 0.2868778675745010664 ) ) ;
#19671=ADVANCED_FACE ( 'NONE', ( #18545 ), #16581, .F. ) ;
#19692=DIRECTION ( 'NONE',  ( -0.2868778675745010664, 0.000000000000000000, -0.9579671649362032637 ) ) ;
#19723=EDGE_CURVE ( 'NONE', #16118, #18438, #8271, .T. ) ;
#19755=DIRECTION ( 'NONE',  ( 0.6050250551579474667, 0.7753173868113220069, -0.1811839737371539749 ) ) ;
#19779=EDGE_CURVE ( 'NONE', #6840, #4597, #10312, .T. ) ;
#19781=CARTESIAN_POINT ( 'NONE',  ( 30.10940225190841701, 2.809619014187358932, -2.349505688218141319 ) ) ;
#19832=VERTEX_POINT ( 'NONE', #10585 ) ;
#19843=CYLINDRICAL_SURFACE ( 'NONE', #5022, 0.7950199999999990608 ) ;
#19862=ORIENTED_EDGE ( 'NONE', *, *, #17647, .F. ) ;
#19864=FACE_OUTER_BOUND ( 'NONE', #4707, .T. ) ;
#19870=CARTESIAN_POINT ( 'NONE',  ( 13.64200589084435578, -5.959792500000001603, -0.3187768451312169571 ) ) ;
#19877=VECTOR ( 'NONE', #4067, 1000.000000000000227 ) ;
#19886=ORIENTED_EDGE ( 'NONE', *, *, #20797, .F. ) ;
#19918=VECTOR ( 'NONE', #4682, 1000.000000000000227 ) ;
#19938=CARTESIAN_POINT ( 'NONE',  ( 13.64200589084435578, -6.754812500000002551, -0.3187768451312169571 ) ) ;
#20004=CARTESIAN_POINT ( 'NONE',  ( 13.67756757867809725, 38.48766750000000059, 2.571257636385987144 ) ) ;
#20009=VERTEX_POINT ( 'NONE', #8100 ) ;
#20087=ORIENTED_EDGE ( 'NONE', *, *, #20399, .F. ) ;
#20119=ADVANCED_FACE ( 'NONE', ( #12093 ), #15529, .T. ) ;
#20127=CYLINDRICAL_SURFACE ( 'NONE', #4415, 0.7950200000000005041 ) ;
#20144=ORIENTED_EDGE ( 'NONE', *, *, #7042, .F. ) ;
#20159=EDGE_LOOP ( 'NONE', ( #12349, #17425, #2642, #2377 ) ) ;
#20179=EDGE_CURVE ( 'NONE', #17126, #3519, #16532, .T. ) ;
#20183=CIRCLE ( 'NONE', #21258, 0.7950199999999990608 ) ;
#20195=DIRECTION ( 'NONE',  ( -0.2868778675745010664, 0.000000000000000000, -0.9579671649362032637 ) ) ;
#20201=ORIENTED_EDGE ( 'NONE', *, *, #13070, .F. ) ;
#20254=( NAMED_UNIT ( * ) PLANE_ANGLE_UNIT ( ) SI_UNIT ( $, .RADIAN. ) );
#20266=DIRECTION ( 'NONE',  ( 0.000000000000000000, -1.000000000000000000, 0.000000000000000000 ) ) ;
#20297=LINE ( 'NONE', #3516, #7741 ) ;
#20305=VECTOR ( 'NONE', #6885, 1000.000000000000000 ) ;
#20313=LINE ( 'NONE', #5182, #21676 ) ;
#20399=EDGE_CURVE ( 'NONE', #10623, #4759, #21629, .T. ) ;
#20424=DIRECTION ( 'NONE',  ( 0.000000000000000000, -1.000000000000000000, 0.000000000000000000 ) ) ;
#20433=CARTESIAN_POINT ( 'NONE',  ( 30.78626241496060700, -5.959792500000001603, -2.552201779827368622 ) ) ;
#20455=EDGE_CURVE ( 'NONE', #21745, #21204, #5042, .T. ) ;
#20468=PRODUCT_CONTEXT ( 'NONE', #16121, 'mechanical' ) ;
#20494=DIRECTION ( 'NONE',  ( -0.2868778675745010664, 0.000000000000000000, -0.9579671649362032637 ) ) ;
#20514=CARTESIAN_POINT ( 'NONE',  ( 30.02465935949302533, 39.28268749999999443, -2.324128137548288731 ) ) ;
#20529=VERTEX_POINT ( 'NONE', #17132 ) ;
#20532=CIRCLE ( 'NONE', #2553, 0.7950199999999993938 ) ;
#20533=EDGE_LOOP ( 'NONE', ( #15483, #4673, #9821, #3636, #5780, #87 ) ) ;
#20555=CARTESIAN_POINT ( 'NONE',  ( 15.47835459351327714, 38.48766750000000059, 5.813316144137728791 ) ) ;
#20569=PLANE ( 'NONE',  #21292 ) ;
#20616=ADVANCED_FACE ( 'NONE', ( #11209 ), #6562, .T. ) ;
#20620=DIRECTION ( 'NONE',  ( -0.2868778675745010664, 0.000000000000000000, -0.9579671649362032637 ) ) ;
#20629=DIRECTION ( 'NONE',  ( -0.2868778675745011220, 0.000000000000000000, -0.9579671649362034858 ) ) ;
#20633=EDGE_LOOP ( 'NONE', ( #285, #8157, #1986, #11324 ) ) ;
#20661=VERTEX_POINT ( 'NONE', #21679 ) ;
#20668=FACE_OUTER_BOUND ( 'NONE', #14642, .T. ) ;
#20671=CARTESIAN_POINT ( 'NONE',  ( 24.43309469626978725, 9.340595522457139310, -0.6496488801123181389 ) ) ;
#20700=AXIS2_PLACEMENT_3D ( 'NONE', #886, #7407, #14181 ) ;
#20727=DIRECTION ( 'NONE',  ( -0.2868778675745010664, 0.000000000000000000, -0.9579671649362032637 ) ) ;
#20741=EDGE_CURVE ( 'NONE', #4404, #12549, #6962, .T. ) ;
#20761=CYLINDRICAL_SURFACE ( 'NONE', #3971, 0.7950200000000005041 ) ;
#20766=ORIENTED_EDGE ( 'NONE', *, *, #20741, .F. ) ;
#20772=EDGE_CURVE ( 'NONE', #21204, #21133, #6632, .T. ) ;
#20797=EDGE_CURVE ( 'NONE', #20661, #1499, #9955, .T. ) ;
#20840=ORIENTED_EDGE ( 'NONE', *, *, #16168, .T. ) ;
#20841=LINE ( 'NONE', #847, #8907 ) ;
#20890=AXIS2_PLACEMENT_3D ( 'NONE', #2857, #14711, #18000 ) ;
#20937=ORIENTED_EDGE ( 'NONE', *, *, #10760, .F. ) ;
#20986=VECTOR ( 'NONE', #6897, 1000.000000000000000 ) ;
#21004=ORIENTED_EDGE ( 'NONE', *, *, #19607, .F. ) ;
#21082=ORIENTED_EDGE ( 'NONE', *, *, #10980, .F. ) ;
#21120=DIRECTION ( 'NONE',  ( -0.2868778675745010664, 0.000000000000000000, -0.9579671649362032637 ) ) ;
#21133=VERTEX_POINT ( 'NONE', #2168 ) ;
#21150=EDGE_CURVE ( 'NONE', #367, #19423, #20841, .T. ) ;
#21164=CARTESIAN_POINT ( 'NONE',  ( 22.04181838752732148, 16.26393749999999727, 0.06645525512612464325 ) ) ;
#21167=FACE_OUTER_BOUND ( 'NONE', #20633, .T. ) ;
#21168=ORIENTED_EDGE ( 'NONE', *, *, #17042, .T. ) ;
#21180=CIRCLE ( 'NONE', #18025, 6.350000000000002309 ) ;
#21191=AXIS2_PLACEMENT_3D ( 'NONE', #10079, #123, #13408 ) ;
#21204=VERTEX_POINT ( 'NONE', #3950 ) ;
#21208=DIRECTION ( 'NONE',  ( -0.2868778675745011220, 0.000000000000000000, -0.9579671649362034858 ) ) ;
#21246=ORIENTED_EDGE ( 'NONE', *, *, #3995, .T. ) ;
#21258=AXIS2_PLACEMENT_3D ( 'NONE', #16582, #21208, #11157 ) ;
#21292=AXIS2_PLACEMENT_3D ( 'NONE', #12634, #679, #5539 ) ;
#21310=CARTESIAN_POINT ( 'NONE',  ( 2.651964239740473683, 13.08893749999999834, 5.873042593501262232 ) ) ;
#21313=CARTESIAN_POINT ( 'NONE',  ( 29.22749461619170219, 39.28268749999999443, -4.986088976786413163 ) ) ;
#21378=ORIENTED_EDGE ( 'NONE', *, *, #7960, .T. ) ;
#21419=CARTESIAN_POINT ( 'NONE',  ( 23.63592995296846766, 9.340595522457139310, -3.311609719350443015 ) ) ;
#21427=DIRECTION ( 'NONE',  ( -0.2868778675745011220, 0.000000000000000000, -0.9579671649362034858 ) ) ;
#21432=VECTOR ( 'NONE', #1847, 1000.000000000000000 ) ;
#21500=VECTOR ( 'NONE', #19692, 1000.000000000000227 ) ;
#21521=ADVANCED_FACE ( 'NONE', ( #2804 ), #14765, .F. ) ;
#21529=DIRECTION ( 'NONE',  ( 0.9579671649362033747, 0.000000000000000000, -0.2868778675745011220 ) ) ;
#21548=EDGE_CURVE ( 'NONE', #16568, #14728, #4574, .T. ) ;
#21561=DIRECTION ( 'NONE',  ( 0.2868778675745011220, 0.000000000000000000, 0.9579671649362034858 ) ) ;
#21626=CARTESIAN_POINT ( 'NONE',  ( 24.71252020198295085, 23.75961143032650114, -0.7333271064221494884 ) ) ;
#21629=CIRCLE ( 'NONE', #5379, 8.929687500000000000 ) ;
#21634=ORIENTED_EDGE ( 'NONE', *, *, #12944, .F. ) ;
#21638=ORIENTED_EDGE ( 'NONE', *, *, #19401, .F. ) ;
#21646=DIRECTION ( 'NONE',  ( 0.2868778675745010664, 0.000000000000000000, 0.9579671649362032637 ) ) ;
#21647=PLANE ( 'NONE',  #11478 ) ;
#21657=ORIENTED_EDGE ( 'NONE', *, *, #8046, .T. ) ;
#21676=VECTOR ( 'NONE', #10391, 1000.000000000000227 ) ;
#21679=CARTESIAN_POINT ( 'NONE',  ( 13.67756757867809725, 1.982787499999999481, 2.571257636385987144 ) ) ;
#21698=VECTOR ( 'NONE', #760, 1000.000000000000000 ) ;
#21710=ORIENTED_EDGE ( 'NONE', *, *, #419, .T. ) ;
#21727=VERTEX_POINT ( 'NONE', #13750 ) ;
#21745=VERTEX_POINT ( 'NONE', #130 ) ;
#21757=CARTESIAN_POINT ( 'NONE',  ( 30.78626241496060700, 30.50833916023545811, -2.552201779827368622 ) ) ;
#21826=ADVANCED_FACE ( 'NONE', ( #7322 ), #20569, .T. ) ;
#21829=EDGE_LOOP ( 'NONE', ( #961, #14802, #11439, #8756, #15710, #10235 ) ) ;
#21844=CARTESIAN_POINT ( 'NONE',  ( 29.22749461619170219, 38.48766750000000059, -4.986088976786413163 ) ) ;
#21871=CARTESIAN_POINT ( 'NONE',  ( 12.88040283537677588, 19.43893749999999798, -0.09070320285213756550 ) ) ;
ENDSEC;
END-ISO-10303-21;
